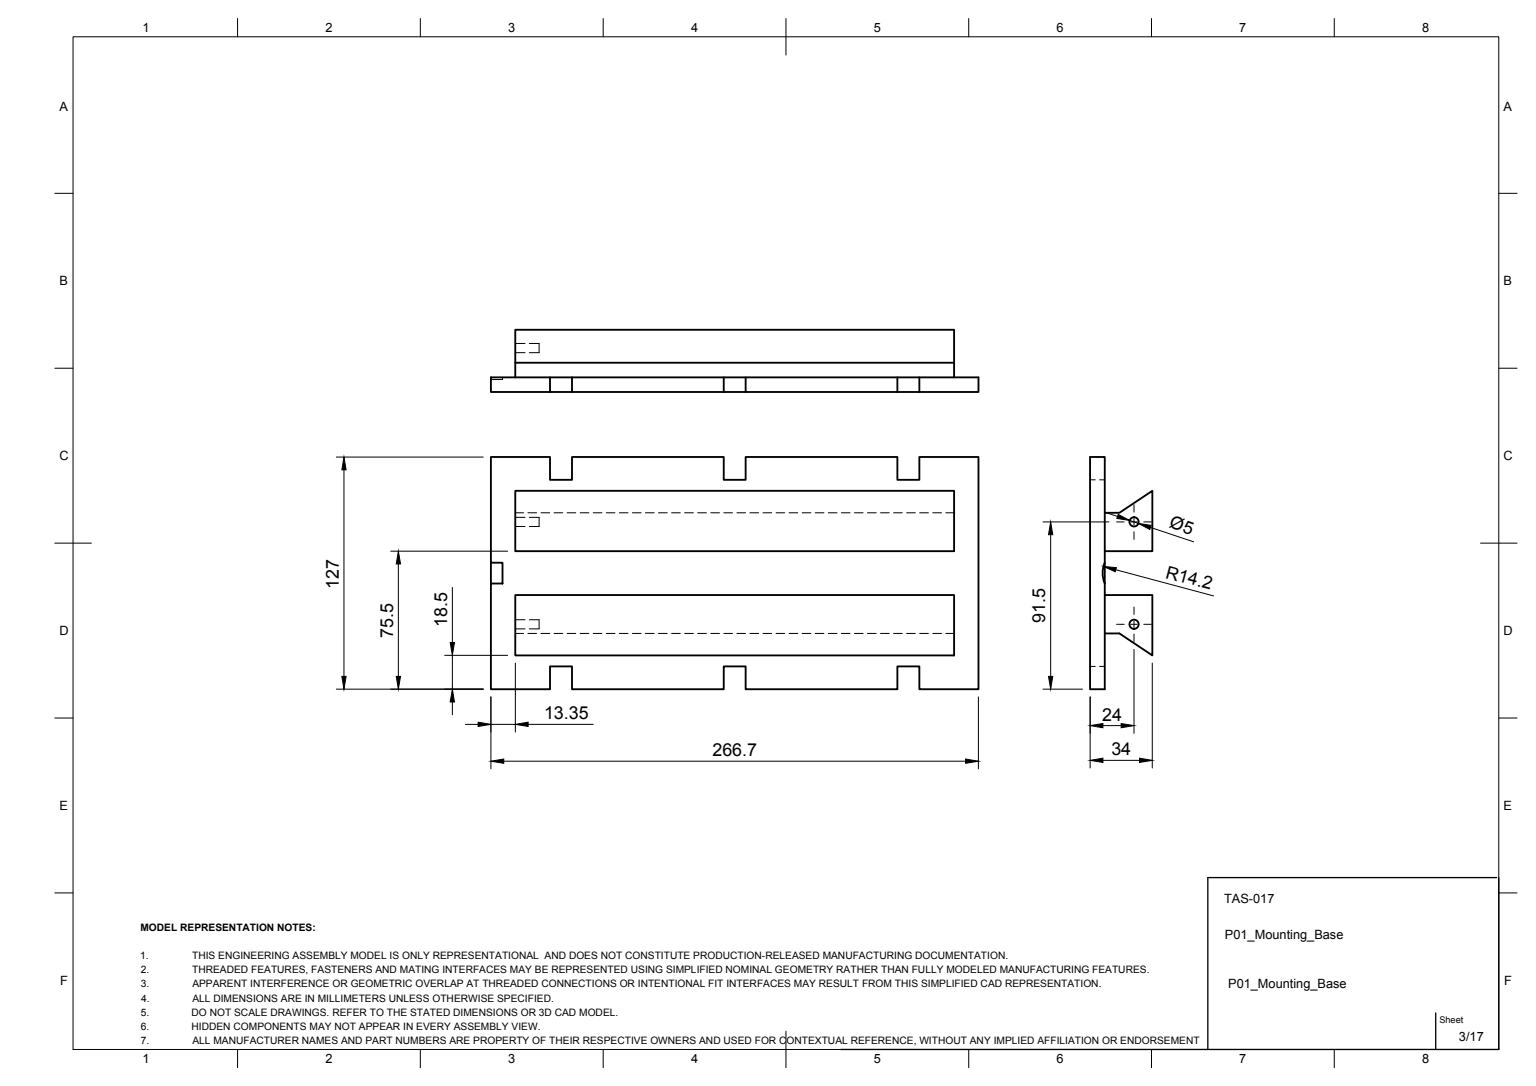
ISO-10303-21;
HEADER;
/* Generated by software containing ST-Developer
 * from STEP Tools, Inc. (www.steptools.com) 
 */

FILE_DESCRIPTION(
/* description */ ('STEP AP203'),
/* implementation_level */ '2;1');

FILE_NAME(
/* name */ 'P01_Mounting_Base.step',
/* time_stamp */ '2026-11-15T15:04:01-08:00',
/* author */ (''),
/* organization */ (''),
/* preprocessor_version */ 'ST-DEVELOPER v20.2',
/* originating_system */ 'Autodesk Translation Framework v15.17.0.0',
/* authorisation */ '');

FILE_SCHEMA (('AUTOMOTIVE_DESIGN { 1 0 10303 214 3 1 1 }'));
ENDSEC;

DATA;
#10=MECHANICAL_DESIGN_GEOMETRIC_PRESENTATION_REPRESENTATION('',(#276,#277,#278),#16598);
#204=SHAPE_REPRESENTATION_RELATIONSHIP('SRR','None',#16698,#228);
#228=ADVANCED_BREP_SHAPE_REPRESENTATION('',(#252),#16574);
#252=MANIFOLD_SOLID_BREP('Body1',#9787);
#276=STYLED_ITEM('',(#16828),#9252);
#277=STYLED_ITEM('',(#16828),#9258);
#278=STYLED_ITEM('',(#16827),#252);
#306=FACE_BOUND('',#1465,.T.);
#307=FACE_BOUND('',#1466,.T.);
#308=FACE_BOUND('',#1484,.T.);
#309=FACE_BOUND('',#1491,.T.);
#429=PLANE('',#10084);
#430=PLANE('',#10085);
#431=PLANE('',#10086);
#432=PLANE('',#10087);
#433=PLANE('',#10088);
#434=PLANE('',#10089);
#435=PLANE('',#10090);
#436=PLANE('',#10091);
#437=PLANE('',#10092);
#438=PLANE('',#10093);
#439=PLANE('',#10094);
#440=PLANE('',#10095);
#441=PLANE('',#10097);
#442=PLANE('',#10098);
#443=PLANE('',#10099);
#444=PLANE('',#10100);
#445=PLANE('',#10101);
#446=PLANE('',#10102);
#447=PLANE('',#10103);
#448=PLANE('',#10104);
#449=PLANE('',#10105);
#450=PLANE('',#10106);
#451=PLANE('',#10107);
#452=PLANE('',#10108);
#453=PLANE('',#10109);
#454=PLANE('',#10110);
#455=PLANE('',#10111);
#456=PLANE('',#10112);
#457=PLANE('',#10113);
#458=PLANE('',#10114);
#459=PLANE('',#10115);
#460=PLANE('',#10116);
#461=PLANE('',#10117);
#462=PLANE('',#10118);
#463=PLANE('',#10119);
#464=PLANE('',#10120);
#465=PLANE('',#10121);
#466=PLANE('',#10122);
#467=PLANE('',#10123);
#468=PLANE('',#10124);
#469=PLANE('',#10125);
#470=PLANE('',#10126);
#471=PLANE('',#10127);
#472=PLANE('',#10128);
#473=PLANE('',#10129);
#911=FACE_OUTER_BOUND('',#1462,.T.);
#912=FACE_OUTER_BOUND('',#1463,.T.);
#913=FACE_OUTER_BOUND('',#1464,.T.);
#914=FACE_OUTER_BOUND('',#1467,.T.);
#915=FACE_OUTER_BOUND('',#1468,.T.);
#916=FACE_OUTER_BOUND('',#1469,.T.);
#917=FACE_OUTER_BOUND('',#1470,.T.);
#918=FACE_OUTER_BOUND('',#1471,.T.);
#919=FACE_OUTER_BOUND('',#1472,.T.);
#920=FACE_OUTER_BOUND('',#1473,.T.);
#921=FACE_OUTER_BOUND('',#1474,.T.);
#922=FACE_OUTER_BOUND('',#1475,.T.);
#923=FACE_OUTER_BOUND('',#1476,.T.);
#924=FACE_OUTER_BOUND('',#1477,.T.);
#925=FACE_OUTER_BOUND('',#1478,.T.);
#926=FACE_OUTER_BOUND('',#1479,.T.);
#927=FACE_OUTER_BOUND('',#1480,.T.);
#928=FACE_OUTER_BOUND('',#1481,.T.);
#929=FACE_OUTER_BOUND('',#1482,.T.);
#930=FACE_OUTER_BOUND('',#1483,.T.);
#931=FACE_OUTER_BOUND('',#1485,.T.);
#932=FACE_OUTER_BOUND('',#1486,.T.);
#933=FACE_OUTER_BOUND('',#1487,.T.);
#934=FACE_OUTER_BOUND('',#1488,.T.);
#935=FACE_OUTER_BOUND('',#1489,.T.);
#936=FACE_OUTER_BOUND('',#1490,.T.);
#937=FACE_OUTER_BOUND('',#1492,.T.);
#938=FACE_OUTER_BOUND('',#1493,.T.);
#939=FACE_OUTER_BOUND('',#1494,.T.);
#940=FACE_OUTER_BOUND('',#1495,.T.);
#941=FACE_OUTER_BOUND('',#1496,.T.);
#942=FACE_OUTER_BOUND('',#1497,.T.);
#943=FACE_OUTER_BOUND('',#1498,.T.);
#944=FACE_OUTER_BOUND('',#1499,.T.);
#945=FACE_OUTER_BOUND('',#1500,.T.);
#946=FACE_OUTER_BOUND('',#1501,.T.);
#947=FACE_OUTER_BOUND('',#1502,.T.);
#948=FACE_OUTER_BOUND('',#1503,.T.);
#949=FACE_OUTER_BOUND('',#1504,.T.);
#950=FACE_OUTER_BOUND('',#1505,.T.);
#951=FACE_OUTER_BOUND('',#1506,.T.);
#952=FACE_OUTER_BOUND('',#1507,.T.);
#953=FACE_OUTER_BOUND('',#1508,.T.);
#954=FACE_OUTER_BOUND('',#1509,.T.);
#955=FACE_OUTER_BOUND('',#1510,.T.);
#956=FACE_OUTER_BOUND('',#1511,.T.);
#957=FACE_OUTER_BOUND('',#1512,.T.);
#958=FACE_OUTER_BOUND('',#1513,.T.);
#1462=EDGE_LOOP('',(#6597,#6598,#6599,#6600));
#1463=EDGE_LOOP('',(#6601,#6602,#6603,#6604));
#1464=EDGE_LOOP('',(#6605,#6606,#6607,#6608,#6609,#6610,#6611,#6612,#6613,
#6614,#6615,#6616,#6617,#6618,#6619,#6620,#6621,#6622,#6623,#6624,#6625,
#6626,#6627,#6628,#6629,#6630,#6631,#6632,#6633,#6634,#6635,#6636));
#1465=EDGE_LOOP('',(#6637,#6638,#6639,#6640));
#1466=EDGE_LOOP('',(#6641,#6642,#6643,#6644));
#1467=EDGE_LOOP('',(#6645,#6646,#6647,#6648));
#1468=EDGE_LOOP('',(#6649,#6650,#6651,#6652));
#1469=EDGE_LOOP('',(#6653,#6654,#6655,#6656));
#1470=EDGE_LOOP('',(#6657,#6658,#6659,#6660));
#1471=EDGE_LOOP('',(#6661,#6662,#6663,#6664));
#1472=EDGE_LOOP('',(#6665,#6666,#6667,#6668));
#1473=EDGE_LOOP('',(#6669,#6670,#6671,#6672));
#1474=EDGE_LOOP('',(#6673,#6674,#6675,#6676));
#1475=EDGE_LOOP('',(#6677,#6678,#6679,#6680,#6681,#6682,#6683,#6684,#6685,
#6686,#6687,#6688,#6689,#6690,#6691,#6692,#6693,#6694,#6695,#6696,#6697,
#6698,#6699,#6700,#6701,#6702,#6703,#6704));
#1476=EDGE_LOOP('',(#6705,#6706,#6707,#6708));
#1477=EDGE_LOOP('',(#6709,#6710,#6711,#6712,#6713,#6714));
#1478=EDGE_LOOP('',(#6715,#6716,#6717,#6718));
#1479=EDGE_LOOP('',(#6719,#6720,#6721,#6722));
#1480=EDGE_LOOP('',(#6723,#6724,#6725,#6726));
#1481=EDGE_LOOP('',(#6727,#6728,#6729,#6730));
#1482=EDGE_LOOP('',(#6731,#6732,#6733,#6734,#6735));
#1483=EDGE_LOOP('',(#6736,#6737,#6738,#6739,#6740));
#1484=EDGE_LOOP('',(#6741));
#1485=EDGE_LOOP('',(#6742,#6743,#6744,#6745));
#1486=EDGE_LOOP('',(#6746,#6747,#6748,#6749));
#1487=EDGE_LOOP('',(#6750,#6751,#6752,#6753));
#1488=EDGE_LOOP('',(#6754,#6755,#6756,#6757));
#1489=EDGE_LOOP('',(#6758,#6759,#6760,#6761,#6762));
#1490=EDGE_LOOP('',(#6763,#6764,#6765,#6766,#6767));
#1491=EDGE_LOOP('',(#6768));
#1492=EDGE_LOOP('',(#6769,#6770,#6771,#6772));
#1493=EDGE_LOOP('',(#6773,#6774,#6775,#6776));
#1494=EDGE_LOOP('',(#6777,#6778,#6779,#6780));
#1495=EDGE_LOOP('',(#6781,#6782,#6783,#6784));
#1496=EDGE_LOOP('',(#6785,#6786,#6787,#6788));
#1497=EDGE_LOOP('',(#6789,#6790,#6791,#6792));
#1498=EDGE_LOOP('',(#6793,#6794,#6795,#6796));
#1499=EDGE_LOOP('',(#6797,#6798,#6799,#6800));
#1500=EDGE_LOOP('',(#6801,#6802,#6803,#6804));
#1501=EDGE_LOOP('',(#6805,#6806,#6807,#6808));
#1502=EDGE_LOOP('',(#6809,#6810,#6811,#6812));
#1503=EDGE_LOOP('',(#6813,#6814,#6815,#6816));
#1504=EDGE_LOOP('',(#6817,#6818,#6819,#6820));
#1505=EDGE_LOOP('',(#6821,#6822,#6823,#6824));
#1506=EDGE_LOOP('',(#6825,#6826,#6827,#6828));
#1507=EDGE_LOOP('',(#6829,#6830,#6831,#6832));
#1508=EDGE_LOOP('',(#6833,#6834,#6835,#6836));
#1509=EDGE_LOOP('',(#6837,#6838,#6839,#6840));
#1510=EDGE_LOOP('',(#6841));
#1511=EDGE_LOOP('',(#6842));
#1512=EDGE_LOOP('',(#6843,#6844));
#1513=EDGE_LOOP('',(#6845,#6846,#6847,#6848));
#2136=LINE('',#13686,#3184);
#2137=LINE('',#13692,#3185);
#2138=LINE('',#13697,#3186);
#2139=LINE('',#13699,#3187);
#2140=LINE('',#13701,#3188);
#2141=LINE('',#13703,#3189);
#2142=LINE('',#13705,#3190);
#2143=LINE('',#13707,#3191);
#2144=LINE('',#13709,#3192);
#2145=LINE('',#13711,#3193);
#2146=LINE('',#13713,#3194);
#2147=LINE('',#13715,#3195);
#2148=LINE('',#13717,#3196);
#2149=LINE('',#13719,#3197);
#2150=LINE('',#13721,#3198);
#2151=LINE('',#13723,#3199);
#2152=LINE('',#13725,#3200);
#2153=LINE('',#13727,#3201);
#2154=LINE('',#13729,#3202);
#2155=LINE('',#13731,#3203);
#2156=LINE('',#13733,#3204);
#2157=LINE('',#13735,#3205);
#2158=LINE('',#13737,#3206);
#2159=LINE('',#13739,#3207);
#2160=LINE('',#13741,#3208);
#2161=LINE('',#13743,#3209);
#2162=LINE('',#13745,#3210);
#2163=LINE('',#13747,#3211);
#2164=LINE('',#13749,#3212);
#2165=LINE('',#13751,#3213);
#2166=LINE('',#13753,#3214);
#2167=LINE('',#13755,#3215);
#2168=LINE('',#13757,#3216);
#2169=LINE('',#13758,#3217);
#2170=LINE('',#13761,#3218);
#2171=LINE('',#13763,#3219);
#2172=LINE('',#13765,#3220);
#2173=LINE('',#13766,#3221);
#2174=LINE('',#13769,#3222);
#2175=LINE('',#13771,#3223);
#2176=LINE('',#13773,#3224);
#2177=LINE('',#13774,#3225);
#2178=LINE('',#13777,#3226);
#2179=LINE('',#13779,#3227);
#2180=LINE('',#13780,#3228);
#2181=LINE('',#13783,#3229);
#2182=LINE('',#13785,#3230);
#2183=LINE('',#13786,#3231);
#2184=LINE('',#13789,#3232);
#2185=LINE('',#13791,#3233);
#2186=LINE('',#13792,#3234);
#2187=LINE('',#13795,#3235);
#2188=LINE('',#13797,#3236);
#2189=LINE('',#13798,#3237);
#2190=LINE('',#13801,#3238);
#2191=LINE('',#13803,#3239);
#2192=LINE('',#13804,#3240);
#2193=LINE('',#13807,#3241);
#2194=LINE('',#13809,#3242);
#2195=LINE('',#13810,#3243);
#2196=LINE('',#13813,#3244);
#2197=LINE('',#13815,#3245);
#2198=LINE('',#13816,#3246);
#2199=LINE('',#13819,#3247);
#2200=LINE('',#13821,#3248);
#2201=LINE('',#13822,#3249);
#2202=LINE('',#13825,#3250);
#2203=LINE('',#13827,#3251);
#2204=LINE('',#13828,#3252);
#2205=LINE('',#13830,#3253);
#2206=LINE('',#13832,#3254);
#2207=LINE('',#13833,#3255);
#2208=LINE('',#13835,#3256);
#2209=LINE('',#13837,#3257);
#2210=LINE('',#13838,#3258);
#2211=LINE('',#13839,#3259);
#2212=LINE('',#13841,#3260);
#2213=LINE('',#13843,#3261);
#2214=LINE('',#13844,#3262);
#2215=LINE('',#13846,#3263);
#2216=LINE('',#13848,#3264);
#2217=LINE('',#13849,#3265);
#2218=LINE('',#13851,#3266);
#2219=LINE('',#13853,#3267);
#2220=LINE('',#13854,#3268);
#2221=LINE('',#13855,#3269);
#2222=LINE('',#13861,#3270);
#2223=LINE('',#13863,#3271);
#2224=LINE('',#13864,#3272);
#2225=LINE('',#13867,#3273);
#2226=LINE('',#13869,#3274);
#2227=LINE('',#13870,#3275);
#2228=LINE('',#13873,#3276);
#2229=LINE('',#13875,#3277);
#2230=LINE('',#13876,#3278);
#2231=LINE('',#13878,#3279);
#2232=LINE('',#13879,#3280);
#2233=LINE('',#13884,#3281);
#2234=LINE('',#13886,#3282);
#2235=LINE('',#13887,#3283);
#2236=LINE('',#13890,#3284);
#2237=LINE('',#13892,#3285);
#2238=LINE('',#13893,#3286);
#2239=LINE('',#13896,#3287);
#2240=LINE('',#13898,#3288);
#2241=LINE('',#13899,#3289);
#2242=LINE('',#13901,#3290);
#2243=LINE('',#13902,#3291);
#2244=LINE('',#13906,#3292);
#2245=LINE('',#13908,#3293);
#2246=LINE('',#13911,#3294);
#2247=LINE('',#13913,#3295);
#2248=LINE('',#13916,#3296);
#2249=LINE('',#13918,#3297);
#2250=LINE('',#13921,#3298);
#2251=LINE('',#13923,#3299);
#2252=LINE('',#13926,#3300);
#2253=LINE('',#13928,#3301);
#2254=LINE('',#13931,#3302);
#2255=LINE('',#13933,#3303);
#3184=VECTOR('',#10936,2.5);
#3185=VECTOR('',#10943,2.5);
#3186=VECTOR('',#10948,1000.);
#3187=VECTOR('',#10949,1000.);
#3188=VECTOR('',#10950,1000.);
#3189=VECTOR('',#10951,1000.);
#3190=VECTOR('',#10952,1000.);
#3191=VECTOR('',#10953,1000.);
#3192=VECTOR('',#10954,1000.);
#3193=VECTOR('',#10955,1000.);
#3194=VECTOR('',#10956,1000.);
#3195=VECTOR('',#10957,1000.);
#3196=VECTOR('',#10958,1000.);
#3197=VECTOR('',#10959,1000.);
#3198=VECTOR('',#10960,1000.);
#3199=VECTOR('',#10961,1000.);
#3200=VECTOR('',#10962,1000.);
#3201=VECTOR('',#10963,1000.);
#3202=VECTOR('',#10964,1000.);
#3203=VECTOR('',#10965,1000.);
#3204=VECTOR('',#10966,1000.);
#3205=VECTOR('',#10967,1000.);
#3206=VECTOR('',#10968,1000.);
#3207=VECTOR('',#10969,1000.);
#3208=VECTOR('',#10970,1000.);
#3209=VECTOR('',#10971,1000.);
#3210=VECTOR('',#10972,1000.);
#3211=VECTOR('',#10973,1000.);
#3212=VECTOR('',#10974,1000.);
#3213=VECTOR('',#10975,1000.);
#3214=VECTOR('',#10976,1000.);
#3215=VECTOR('',#10977,1000.);
#3216=VECTOR('',#10978,1000.);
#3217=VECTOR('',#10979,1000.);
#3218=VECTOR('',#10980,1000.);
#3219=VECTOR('',#10981,1000.);
#3220=VECTOR('',#10982,1000.);
#3221=VECTOR('',#10983,1000.);
#3222=VECTOR('',#10984,1000.);
#3223=VECTOR('',#10985,1000.);
#3224=VECTOR('',#10986,1000.);
#3225=VECTOR('',#10987,1000.);
#3226=VECTOR('',#10990,1000.);
#3227=VECTOR('',#10991,1000.);
#3228=VECTOR('',#10992,1000.);
#3229=VECTOR('',#10995,1000.);
#3230=VECTOR('',#10996,1000.);
#3231=VECTOR('',#10997,1000.);
#3232=VECTOR('',#11000,1000.);
#3233=VECTOR('',#11001,1000.);
#3234=VECTOR('',#11002,1000.);
#3235=VECTOR('',#11005,1000.);
#3236=VECTOR('',#11006,1000.);
#3237=VECTOR('',#11007,1000.);
#3238=VECTOR('',#11010,1000.);
#3239=VECTOR('',#11011,1000.);
#3240=VECTOR('',#11012,1000.);
#3241=VECTOR('',#11015,1000.);
#3242=VECTOR('',#11016,1000.);
#3243=VECTOR('',#11017,1000.);
#3244=VECTOR('',#11020,1000.);
#3245=VECTOR('',#11021,1000.);
#3246=VECTOR('',#11022,1000.);
#3247=VECTOR('',#11025,1000.);
#3248=VECTOR('',#11026,1000.);
#3249=VECTOR('',#11027,1000.);
#3250=VECTOR('',#11030,1000.);
#3251=VECTOR('',#11031,1000.);
#3252=VECTOR('',#11032,1000.);
#3253=VECTOR('',#11033,1000.);
#3254=VECTOR('',#11034,1000.);
#3255=VECTOR('',#11035,1000.);
#3256=VECTOR('',#11036,1000.);
#3257=VECTOR('',#11037,1000.);
#3258=VECTOR('',#11038,1000.);
#3259=VECTOR('',#11039,1000.);
#3260=VECTOR('',#11040,1000.);
#3261=VECTOR('',#11041,1000.);
#3262=VECTOR('',#11042,1000.);
#3263=VECTOR('',#11043,1000.);
#3264=VECTOR('',#11044,1000.);
#3265=VECTOR('',#11045,1000.);
#3266=VECTOR('',#11046,1000.);
#3267=VECTOR('',#11047,1000.);
#3268=VECTOR('',#11048,1000.);
#3269=VECTOR('',#11049,1000.);
#3270=VECTOR('',#11058,1000.);
#3271=VECTOR('',#11059,1000.);
#3272=VECTOR('',#11060,1000.);
#3273=VECTOR('',#11063,1000.);
#3274=VECTOR('',#11064,1000.);
#3275=VECTOR('',#11065,1000.);
#3276=VECTOR('',#11068,1000.);
#3277=VECTOR('',#11069,1000.);
#3278=VECTOR('',#11070,1000.);
#3279=VECTOR('',#11073,1000.);
#3280=VECTOR('',#11074,1000.);
#3281=VECTOR('',#11081,1000.);
#3282=VECTOR('',#11082,1000.);
#3283=VECTOR('',#11083,1000.);
#3284=VECTOR('',#11086,1000.);
#3285=VECTOR('',#11087,1000.);
#3286=VECTOR('',#11088,1000.);
#3287=VECTOR('',#11091,1000.);
#3288=VECTOR('',#11092,1000.);
#3289=VECTOR('',#11093,1000.);
#3290=VECTOR('',#11096,1000.);
#3291=VECTOR('',#11097,1000.);
#3292=VECTOR('',#11104,1000.);
#3293=VECTOR('',#11107,1000.);
#3294=VECTOR('',#11112,1000.);
#3295=VECTOR('',#11115,1000.);
#3296=VECTOR('',#11120,1000.);
#3297=VECTOR('',#11123,1000.);
#3298=VECTOR('',#11128,1000.);
#3299=VECTOR('',#11131,1000.);
#3300=VECTOR('',#11136,1000.);
#3301=VECTOR('',#11139,1000.);
#3302=VECTOR('',#11144,1000.);
#3303=VECTOR('',#11147,1000.);
#4232=CIRCLE('',#10079,2.5);
#4233=CIRCLE('',#10080,2.5);
#4234=CIRCLE('',#10082,2.5);
#4235=CIRCLE('',#10083,2.5);
#4236=CIRCLE('',#10096,14.2);
#4237=CIRCLE('',#10130,14.2);
#4455=VERTEX_POINT('',#13683);
#4456=VERTEX_POINT('',#13685);
#4457=VERTEX_POINT('',#13689);
#4458=VERTEX_POINT('',#13691);
#4459=VERTEX_POINT('',#13695);
#4460=VERTEX_POINT('',#13696);
#4461=VERTEX_POINT('',#13698);
#4462=VERTEX_POINT('',#13700);
#4463=VERTEX_POINT('',#13702);
#4464=VERTEX_POINT('',#13704);
#4465=VERTEX_POINT('',#13706);
#4466=VERTEX_POINT('',#13708);
#4467=VERTEX_POINT('',#13710);
#4468=VERTEX_POINT('',#13712);
#4469=VERTEX_POINT('',#13714);
#4470=VERTEX_POINT('',#13716);
#4471=VERTEX_POINT('',#13718);
#4472=VERTEX_POINT('',#13720);
#4473=VERTEX_POINT('',#13722);
#4474=VERTEX_POINT('',#13724);
#4475=VERTEX_POINT('',#13726);
#4476=VERTEX_POINT('',#13728);
#4477=VERTEX_POINT('',#13730);
#4478=VERTEX_POINT('',#13732);
#4479=VERTEX_POINT('',#13734);
#4480=VERTEX_POINT('',#13736);
#4481=VERTEX_POINT('',#13738);
#4482=VERTEX_POINT('',#13740);
#4483=VERTEX_POINT('',#13742);
#4484=VERTEX_POINT('',#13744);
#4485=VERTEX_POINT('',#13746);
#4486=VERTEX_POINT('',#13748);
#4487=VERTEX_POINT('',#13750);
#4488=VERTEX_POINT('',#13752);
#4489=VERTEX_POINT('',#13754);
#4490=VERTEX_POINT('',#13756);
#4491=VERTEX_POINT('',#13759);
#4492=VERTEX_POINT('',#13760);
#4493=VERTEX_POINT('',#13762);
#4494=VERTEX_POINT('',#13764);
#4495=VERTEX_POINT('',#13767);
#4496=VERTEX_POINT('',#13768);
#4497=VERTEX_POINT('',#13770);
#4498=VERTEX_POINT('',#13772);
#4499=VERTEX_POINT('',#13776);
#4500=VERTEX_POINT('',#13778);
#4501=VERTEX_POINT('',#13782);
#4502=VERTEX_POINT('',#13784);
#4503=VERTEX_POINT('',#13788);
#4504=VERTEX_POINT('',#13790);
#4505=VERTEX_POINT('',#13794);
#4506=VERTEX_POINT('',#13796);
#4507=VERTEX_POINT('',#13800);
#4508=VERTEX_POINT('',#13802);
#4509=VERTEX_POINT('',#13806);
#4510=VERTEX_POINT('',#13808);
#4511=VERTEX_POINT('',#13812);
#4512=VERTEX_POINT('',#13814);
#4513=VERTEX_POINT('',#13818);
#4514=VERTEX_POINT('',#13820);
#4515=VERTEX_POINT('',#13824);
#4516=VERTEX_POINT('',#13826);
#4517=VERTEX_POINT('',#13829);
#4518=VERTEX_POINT('',#13831);
#4519=VERTEX_POINT('',#13834);
#4520=VERTEX_POINT('',#13836);
#4521=VERTEX_POINT('',#13840);
#4522=VERTEX_POINT('',#13842);
#4523=VERTEX_POINT('',#13845);
#4524=VERTEX_POINT('',#13847);
#4525=VERTEX_POINT('',#13850);
#4526=VERTEX_POINT('',#13852);
#4527=VERTEX_POINT('',#13860);
#4528=VERTEX_POINT('',#13862);
#4529=VERTEX_POINT('',#13866);
#4530=VERTEX_POINT('',#13868);
#4531=VERTEX_POINT('',#13872);
#4532=VERTEX_POINT('',#13874);
#4533=VERTEX_POINT('',#13883);
#4534=VERTEX_POINT('',#13885);
#4535=VERTEX_POINT('',#13889);
#4536=VERTEX_POINT('',#13891);
#4537=VERTEX_POINT('',#13895);
#4538=VERTEX_POINT('',#13897);
#5311=EDGE_CURVE('',#4455,#4455,#4232,.T.);
#5312=EDGE_CURVE('',#4455,#4456,#2136,.T.);
#5313=EDGE_CURVE('',#4456,#4456,#4233,.T.);
#5314=EDGE_CURVE('',#4457,#4457,#4234,.T.);
#5315=EDGE_CURVE('',#4457,#4458,#2137,.T.);
#5316=EDGE_CURVE('',#4458,#4458,#4235,.T.);
#5317=EDGE_CURVE('',#4459,#4460,#2138,.T.);
#5318=EDGE_CURVE('',#4459,#4461,#2139,.T.);
#5319=EDGE_CURVE('',#4461,#4462,#2140,.T.);
#5320=EDGE_CURVE('',#4463,#4462,#2141,.T.);
#5321=EDGE_CURVE('',#4464,#4463,#2142,.T.);
#5322=EDGE_CURVE('',#4465,#4464,#2143,.T.);
#5323=EDGE_CURVE('',#4465,#4466,#2144,.T.);
#5324=EDGE_CURVE('',#4467,#4466,#2145,.T.);
#5325=EDGE_CURVE('',#4468,#4467,#2146,.T.);
#5326=EDGE_CURVE('',#4469,#4468,#2147,.T.);
#5327=EDGE_CURVE('',#4469,#4470,#2148,.T.);
#5328=EDGE_CURVE('',#4471,#4470,#2149,.T.);
#5329=EDGE_CURVE('',#4472,#4471,#2150,.T.);
#5330=EDGE_CURVE('',#4473,#4472,#2151,.T.);
#5331=EDGE_CURVE('',#4473,#4474,#2152,.T.);
#5332=EDGE_CURVE('',#4474,#4475,#2153,.T.);
#5333=EDGE_CURVE('',#4475,#4476,#2154,.T.);
#5334=EDGE_CURVE('',#4477,#4476,#2155,.T.);
#5335=EDGE_CURVE('',#4478,#4477,#2156,.T.);
#5336=EDGE_CURVE('',#4479,#4478,#2157,.T.);
#5337=EDGE_CURVE('',#4479,#4480,#2158,.T.);
#5338=EDGE_CURVE('',#4481,#4480,#2159,.T.);
#5339=EDGE_CURVE('',#4482,#4481,#2160,.T.);
#5340=EDGE_CURVE('',#4483,#4482,#2161,.T.);
#5341=EDGE_CURVE('',#4483,#4484,#2162,.T.);
#5342=EDGE_CURVE('',#4485,#4484,#2163,.T.);
#5343=EDGE_CURVE('',#4486,#4485,#2164,.T.);
#5344=EDGE_CURVE('',#4487,#4486,#2165,.T.);
#5345=EDGE_CURVE('',#4487,#4488,#2166,.T.);
#5346=EDGE_CURVE('',#4488,#4489,#2167,.T.);
#5347=EDGE_CURVE('',#4490,#4489,#2168,.T.);
#5348=EDGE_CURVE('',#4490,#4460,#2169,.T.);
#5349=EDGE_CURVE('',#4491,#4492,#2170,.T.);
#5350=EDGE_CURVE('',#4491,#4493,#2171,.T.);
#5351=EDGE_CURVE('',#4493,#4494,#2172,.T.);
#5352=EDGE_CURVE('',#4492,#4494,#2173,.T.);
#5353=EDGE_CURVE('',#4495,#4496,#2174,.T.);
#5354=EDGE_CURVE('',#4497,#4495,#2175,.T.);
#5355=EDGE_CURVE('',#4497,#4498,#2176,.T.);
#5356=EDGE_CURVE('',#4498,#4496,#2177,.T.);
#5357=EDGE_CURVE('',#4480,#4499,#2178,.T.);
#5358=EDGE_CURVE('',#4500,#4479,#2179,.T.);
#5359=EDGE_CURVE('',#4500,#4499,#2180,.T.);
#5360=EDGE_CURVE('',#4501,#4483,#2181,.T.);
#5361=EDGE_CURVE('',#4501,#4502,#2182,.T.);
#5362=EDGE_CURVE('',#4484,#4502,#2183,.T.);
#5363=EDGE_CURVE('',#4503,#4487,#2184,.T.);
#5364=EDGE_CURVE('',#4503,#4504,#2185,.T.);
#5365=EDGE_CURVE('',#4488,#4504,#2186,.T.);
#5366=EDGE_CURVE('',#4476,#4505,#2187,.T.);
#5367=EDGE_CURVE('',#4475,#4506,#2188,.T.);
#5368=EDGE_CURVE('',#4506,#4505,#2189,.T.);
#5369=EDGE_CURVE('',#4507,#4473,#2190,.T.);
#5370=EDGE_CURVE('',#4507,#4508,#2191,.T.);
#5371=EDGE_CURVE('',#4474,#4508,#2192,.T.);
#5372=EDGE_CURVE('',#4470,#4509,#2193,.T.);
#5373=EDGE_CURVE('',#4510,#4469,#2194,.T.);
#5374=EDGE_CURVE('',#4510,#4509,#2195,.T.);
#5375=EDGE_CURVE('',#4466,#4511,#2196,.T.);
#5376=EDGE_CURVE('',#4512,#4465,#2197,.T.);
#5377=EDGE_CURVE('',#4512,#4511,#2198,.T.);
#5378=EDGE_CURVE('',#4462,#4513,#2199,.T.);
#5379=EDGE_CURVE('',#4461,#4514,#2200,.T.);
#5380=EDGE_CURVE('',#4514,#4513,#2201,.T.);
#5381=EDGE_CURVE('',#4507,#4515,#2202,.T.);
#5382=EDGE_CURVE('',#4515,#4516,#2203,.T.);
#5383=EDGE_CURVE('',#4516,#4509,#2204,.T.);
#5384=EDGE_CURVE('',#4510,#4517,#2205,.T.);
#5385=EDGE_CURVE('',#4517,#4518,#2206,.T.);
#5386=EDGE_CURVE('',#4518,#4511,#2207,.T.);
#5387=EDGE_CURVE('',#4512,#4519,#2208,.T.);
#5388=EDGE_CURVE('',#4519,#4520,#2209,.T.);
#5389=EDGE_CURVE('',#4520,#4513,#2210,.T.);
#5390=EDGE_CURVE('',#4504,#4514,#2211,.T.);
#5391=EDGE_CURVE('',#4503,#4521,#2212,.T.);
#5392=EDGE_CURVE('',#4521,#4522,#2213,.T.);
#5393=EDGE_CURVE('',#4522,#4502,#2214,.T.);
#5394=EDGE_CURVE('',#4501,#4523,#2215,.T.);
#5395=EDGE_CURVE('',#4523,#4524,#2216,.T.);
#5396=EDGE_CURVE('',#4524,#4499,#2217,.T.);
#5397=EDGE_CURVE('',#4500,#4525,#2218,.T.);
#5398=EDGE_CURVE('',#4525,#4526,#2219,.T.);
#5399=EDGE_CURVE('',#4526,#4505,#2220,.T.);
#5400=EDGE_CURVE('',#4508,#4506,#2221,.T.);
#5401=EDGE_CURVE('',#4489,#4459,#4236,.T.);
#5402=EDGE_CURVE('',#4527,#4498,#2222,.T.);
#5403=EDGE_CURVE('',#4528,#4497,#2223,.T.);
#5404=EDGE_CURVE('',#4528,#4527,#2224,.T.);
#5405=EDGE_CURVE('',#4496,#4529,#2225,.T.);
#5406=EDGE_CURVE('',#4530,#4529,#2226,.T.);
#5407=EDGE_CURVE('',#4495,#4530,#2227,.T.);
#5408=EDGE_CURVE('',#4529,#4531,#2228,.T.);
#5409=EDGE_CURVE('',#4532,#4531,#2229,.T.);
#5410=EDGE_CURVE('',#4530,#4532,#2230,.T.);
#5411=EDGE_CURVE('',#4531,#4527,#2231,.T.);
#5412=EDGE_CURVE('',#4532,#4528,#2232,.T.);
#5413=EDGE_CURVE('',#4494,#4533,#2233,.T.);
#5414=EDGE_CURVE('',#4534,#4533,#2234,.T.);
#5415=EDGE_CURVE('',#4492,#4534,#2235,.T.);
#5416=EDGE_CURVE('',#4533,#4535,#2236,.T.);
#5417=EDGE_CURVE('',#4536,#4535,#2237,.T.);
#5418=EDGE_CURVE('',#4534,#4536,#2238,.T.);
#5419=EDGE_CURVE('',#4535,#4537,#2239,.T.);
#5420=EDGE_CURVE('',#4538,#4537,#2240,.T.);
#5421=EDGE_CURVE('',#4536,#4538,#2241,.T.);
#5422=EDGE_CURVE('',#4537,#4493,#2242,.T.);
#5423=EDGE_CURVE('',#4538,#4491,#2243,.T.);
#5424=EDGE_CURVE('',#4464,#4519,#2244,.T.);
#5425=EDGE_CURVE('',#4463,#4520,#2245,.T.);
#5426=EDGE_CURVE('',#4477,#4526,#2246,.T.);
#5427=EDGE_CURVE('',#4478,#4525,#2247,.T.);
#5428=EDGE_CURVE('',#4485,#4522,#2248,.T.);
#5429=EDGE_CURVE('',#4486,#4521,#2249,.T.);
#5430=EDGE_CURVE('',#4468,#4517,#2250,.T.);
#5431=EDGE_CURVE('',#4467,#4518,#2251,.T.);
#5432=EDGE_CURVE('',#4481,#4524,#2252,.T.);
#5433=EDGE_CURVE('',#4482,#4523,#2253,.T.);
#5434=EDGE_CURVE('',#4472,#4515,#2254,.T.);
#5435=EDGE_CURVE('',#4471,#4516,#2255,.T.);
#5436=EDGE_CURVE('',#4460,#4490,#4237,.T.);
#6597=ORIENTED_EDGE('',*,*,#5311,.T.);
#6598=ORIENTED_EDGE('',*,*,#5312,.T.);
#6599=ORIENTED_EDGE('',*,*,#5313,.T.);
#6600=ORIENTED_EDGE('',*,*,#5312,.F.);
#6601=ORIENTED_EDGE('',*,*,#5314,.T.);
#6602=ORIENTED_EDGE('',*,*,#5315,.T.);
#6603=ORIENTED_EDGE('',*,*,#5316,.F.);
#6604=ORIENTED_EDGE('',*,*,#5315,.F.);
#6605=ORIENTED_EDGE('',*,*,#5317,.F.);
#6606=ORIENTED_EDGE('',*,*,#5318,.T.);
#6607=ORIENTED_EDGE('',*,*,#5319,.T.);
#6608=ORIENTED_EDGE('',*,*,#5320,.F.);
#6609=ORIENTED_EDGE('',*,*,#5321,.F.);
#6610=ORIENTED_EDGE('',*,*,#5322,.F.);
#6611=ORIENTED_EDGE('',*,*,#5323,.T.);
#6612=ORIENTED_EDGE('',*,*,#5324,.F.);
#6613=ORIENTED_EDGE('',*,*,#5325,.F.);
#6614=ORIENTED_EDGE('',*,*,#5326,.F.);
#6615=ORIENTED_EDGE('',*,*,#5327,.T.);
#6616=ORIENTED_EDGE('',*,*,#5328,.F.);
#6617=ORIENTED_EDGE('',*,*,#5329,.F.);
#6618=ORIENTED_EDGE('',*,*,#5330,.F.);
#6619=ORIENTED_EDGE('',*,*,#5331,.T.);
#6620=ORIENTED_EDGE('',*,*,#5332,.T.);
#6621=ORIENTED_EDGE('',*,*,#5333,.T.);
#6622=ORIENTED_EDGE('',*,*,#5334,.F.);
#6623=ORIENTED_EDGE('',*,*,#5335,.F.);
#6624=ORIENTED_EDGE('',*,*,#5336,.F.);
#6625=ORIENTED_EDGE('',*,*,#5337,.T.);
#6626=ORIENTED_EDGE('',*,*,#5338,.F.);
#6627=ORIENTED_EDGE('',*,*,#5339,.F.);
#6628=ORIENTED_EDGE('',*,*,#5340,.F.);
#6629=ORIENTED_EDGE('',*,*,#5341,.T.);
#6630=ORIENTED_EDGE('',*,*,#5342,.F.);
#6631=ORIENTED_EDGE('',*,*,#5343,.F.);
#6632=ORIENTED_EDGE('',*,*,#5344,.F.);
#6633=ORIENTED_EDGE('',*,*,#5345,.T.);
#6634=ORIENTED_EDGE('',*,*,#5346,.T.);
#6635=ORIENTED_EDGE('',*,*,#5347,.F.);
#6636=ORIENTED_EDGE('',*,*,#5348,.T.);
#6637=ORIENTED_EDGE('',*,*,#5349,.F.);
#6638=ORIENTED_EDGE('',*,*,#5350,.T.);
#6639=ORIENTED_EDGE('',*,*,#5351,.T.);
#6640=ORIENTED_EDGE('',*,*,#5352,.F.);
#6641=ORIENTED_EDGE('',*,*,#5353,.F.);
#6642=ORIENTED_EDGE('',*,*,#5354,.F.);
#6643=ORIENTED_EDGE('',*,*,#5355,.T.);
#6644=ORIENTED_EDGE('',*,*,#5356,.T.);
#6645=ORIENTED_EDGE('',*,*,#5357,.F.);
#6646=ORIENTED_EDGE('',*,*,#5337,.F.);
#6647=ORIENTED_EDGE('',*,*,#5358,.F.);
#6648=ORIENTED_EDGE('',*,*,#5359,.T.);
#6649=ORIENTED_EDGE('',*,*,#5360,.F.);
#6650=ORIENTED_EDGE('',*,*,#5361,.T.);
#6651=ORIENTED_EDGE('',*,*,#5362,.F.);
#6652=ORIENTED_EDGE('',*,*,#5341,.F.);
#6653=ORIENTED_EDGE('',*,*,#5363,.F.);
#6654=ORIENTED_EDGE('',*,*,#5364,.T.);
#6655=ORIENTED_EDGE('',*,*,#5365,.F.);
#6656=ORIENTED_EDGE('',*,*,#5345,.F.);
#6657=ORIENTED_EDGE('',*,*,#5366,.F.);
#6658=ORIENTED_EDGE('',*,*,#5333,.F.);
#6659=ORIENTED_EDGE('',*,*,#5367,.T.);
#6660=ORIENTED_EDGE('',*,*,#5368,.T.);
#6661=ORIENTED_EDGE('',*,*,#5369,.F.);
#6662=ORIENTED_EDGE('',*,*,#5370,.T.);
#6663=ORIENTED_EDGE('',*,*,#5371,.F.);
#6664=ORIENTED_EDGE('',*,*,#5331,.F.);
#6665=ORIENTED_EDGE('',*,*,#5372,.F.);
#6666=ORIENTED_EDGE('',*,*,#5327,.F.);
#6667=ORIENTED_EDGE('',*,*,#5373,.F.);
#6668=ORIENTED_EDGE('',*,*,#5374,.T.);
#6669=ORIENTED_EDGE('',*,*,#5375,.F.);
#6670=ORIENTED_EDGE('',*,*,#5323,.F.);
#6671=ORIENTED_EDGE('',*,*,#5376,.F.);
#6672=ORIENTED_EDGE('',*,*,#5377,.T.);
#6673=ORIENTED_EDGE('',*,*,#5378,.F.);
#6674=ORIENTED_EDGE('',*,*,#5319,.F.);
#6675=ORIENTED_EDGE('',*,*,#5379,.T.);
#6676=ORIENTED_EDGE('',*,*,#5380,.T.);
#6677=ORIENTED_EDGE('',*,*,#5370,.F.);
#6678=ORIENTED_EDGE('',*,*,#5381,.T.);
#6679=ORIENTED_EDGE('',*,*,#5382,.T.);
#6680=ORIENTED_EDGE('',*,*,#5383,.T.);
#6681=ORIENTED_EDGE('',*,*,#5374,.F.);
#6682=ORIENTED_EDGE('',*,*,#5384,.T.);
#6683=ORIENTED_EDGE('',*,*,#5385,.T.);
#6684=ORIENTED_EDGE('',*,*,#5386,.T.);
#6685=ORIENTED_EDGE('',*,*,#5377,.F.);
#6686=ORIENTED_EDGE('',*,*,#5387,.T.);
#6687=ORIENTED_EDGE('',*,*,#5388,.T.);
#6688=ORIENTED_EDGE('',*,*,#5389,.T.);
#6689=ORIENTED_EDGE('',*,*,#5380,.F.);
#6690=ORIENTED_EDGE('',*,*,#5390,.F.);
#6691=ORIENTED_EDGE('',*,*,#5364,.F.);
#6692=ORIENTED_EDGE('',*,*,#5391,.T.);
#6693=ORIENTED_EDGE('',*,*,#5392,.T.);
#6694=ORIENTED_EDGE('',*,*,#5393,.T.);
#6695=ORIENTED_EDGE('',*,*,#5361,.F.);
#6696=ORIENTED_EDGE('',*,*,#5394,.T.);
#6697=ORIENTED_EDGE('',*,*,#5395,.T.);
#6698=ORIENTED_EDGE('',*,*,#5396,.T.);
#6699=ORIENTED_EDGE('',*,*,#5359,.F.);
#6700=ORIENTED_EDGE('',*,*,#5397,.T.);
#6701=ORIENTED_EDGE('',*,*,#5398,.T.);
#6702=ORIENTED_EDGE('',*,*,#5399,.T.);
#6703=ORIENTED_EDGE('',*,*,#5368,.F.);
#6704=ORIENTED_EDGE('',*,*,#5400,.F.);
#6705=ORIENTED_EDGE('',*,*,#5400,.T.);
#6706=ORIENTED_EDGE('',*,*,#5367,.F.);
#6707=ORIENTED_EDGE('',*,*,#5332,.F.);
#6708=ORIENTED_EDGE('',*,*,#5371,.T.);
#6709=ORIENTED_EDGE('',*,*,#5401,.F.);
#6710=ORIENTED_EDGE('',*,*,#5346,.F.);
#6711=ORIENTED_EDGE('',*,*,#5365,.T.);
#6712=ORIENTED_EDGE('',*,*,#5390,.T.);
#6713=ORIENTED_EDGE('',*,*,#5379,.F.);
#6714=ORIENTED_EDGE('',*,*,#5318,.F.);
#6715=ORIENTED_EDGE('',*,*,#5402,.T.);
#6716=ORIENTED_EDGE('',*,*,#5355,.F.);
#6717=ORIENTED_EDGE('',*,*,#5403,.F.);
#6718=ORIENTED_EDGE('',*,*,#5404,.T.);
#6719=ORIENTED_EDGE('',*,*,#5405,.T.);
#6720=ORIENTED_EDGE('',*,*,#5406,.F.);
#6721=ORIENTED_EDGE('',*,*,#5407,.F.);
#6722=ORIENTED_EDGE('',*,*,#5353,.T.);
#6723=ORIENTED_EDGE('',*,*,#5408,.T.);
#6724=ORIENTED_EDGE('',*,*,#5409,.F.);
#6725=ORIENTED_EDGE('',*,*,#5410,.F.);
#6726=ORIENTED_EDGE('',*,*,#5406,.T.);
#6727=ORIENTED_EDGE('',*,*,#5411,.T.);
#6728=ORIENTED_EDGE('',*,*,#5404,.F.);
#6729=ORIENTED_EDGE('',*,*,#5412,.F.);
#6730=ORIENTED_EDGE('',*,*,#5409,.T.);
#6731=ORIENTED_EDGE('',*,*,#5403,.T.);
#6732=ORIENTED_EDGE('',*,*,#5354,.T.);
#6733=ORIENTED_EDGE('',*,*,#5407,.T.);
#6734=ORIENTED_EDGE('',*,*,#5410,.T.);
#6735=ORIENTED_EDGE('',*,*,#5412,.T.);
#6736=ORIENTED_EDGE('',*,*,#5402,.F.);
#6737=ORIENTED_EDGE('',*,*,#5411,.F.);
#6738=ORIENTED_EDGE('',*,*,#5408,.F.);
#6739=ORIENTED_EDGE('',*,*,#5405,.F.);
#6740=ORIENTED_EDGE('',*,*,#5356,.F.);
#6741=ORIENTED_EDGE('',*,*,#5313,.F.);
#6742=ORIENTED_EDGE('',*,*,#5413,.T.);
#6743=ORIENTED_EDGE('',*,*,#5414,.F.);
#6744=ORIENTED_EDGE('',*,*,#5415,.F.);
#6745=ORIENTED_EDGE('',*,*,#5352,.T.);
#6746=ORIENTED_EDGE('',*,*,#5416,.T.);
#6747=ORIENTED_EDGE('',*,*,#5417,.F.);
#6748=ORIENTED_EDGE('',*,*,#5418,.F.);
#6749=ORIENTED_EDGE('',*,*,#5414,.T.);
#6750=ORIENTED_EDGE('',*,*,#5419,.T.);
#6751=ORIENTED_EDGE('',*,*,#5420,.F.);
#6752=ORIENTED_EDGE('',*,*,#5421,.F.);
#6753=ORIENTED_EDGE('',*,*,#5417,.T.);
#6754=ORIENTED_EDGE('',*,*,#5422,.T.);
#6755=ORIENTED_EDGE('',*,*,#5350,.F.);
#6756=ORIENTED_EDGE('',*,*,#5423,.F.);
#6757=ORIENTED_EDGE('',*,*,#5420,.T.);
#6758=ORIENTED_EDGE('',*,*,#5415,.T.);
#6759=ORIENTED_EDGE('',*,*,#5418,.T.);
#6760=ORIENTED_EDGE('',*,*,#5421,.T.);
#6761=ORIENTED_EDGE('',*,*,#5423,.T.);
#6762=ORIENTED_EDGE('',*,*,#5349,.T.);
#6763=ORIENTED_EDGE('',*,*,#5413,.F.);
#6764=ORIENTED_EDGE('',*,*,#5351,.F.);
#6765=ORIENTED_EDGE('',*,*,#5422,.F.);
#6766=ORIENTED_EDGE('',*,*,#5419,.F.);
#6767=ORIENTED_EDGE('',*,*,#5416,.F.);
#6768=ORIENTED_EDGE('',*,*,#5316,.T.);
#6769=ORIENTED_EDGE('',*,*,#5322,.T.);
#6770=ORIENTED_EDGE('',*,*,#5424,.T.);
#6771=ORIENTED_EDGE('',*,*,#5387,.F.);
#6772=ORIENTED_EDGE('',*,*,#5376,.T.);
#6773=ORIENTED_EDGE('',*,*,#5321,.T.);
#6774=ORIENTED_EDGE('',*,*,#5425,.T.);
#6775=ORIENTED_EDGE('',*,*,#5388,.F.);
#6776=ORIENTED_EDGE('',*,*,#5424,.F.);
#6777=ORIENTED_EDGE('',*,*,#5320,.T.);
#6778=ORIENTED_EDGE('',*,*,#5378,.T.);
#6779=ORIENTED_EDGE('',*,*,#5389,.F.);
#6780=ORIENTED_EDGE('',*,*,#5425,.F.);
#6781=ORIENTED_EDGE('',*,*,#5334,.T.);
#6782=ORIENTED_EDGE('',*,*,#5366,.T.);
#6783=ORIENTED_EDGE('',*,*,#5399,.F.);
#6784=ORIENTED_EDGE('',*,*,#5426,.F.);
#6785=ORIENTED_EDGE('',*,*,#5336,.T.);
#6786=ORIENTED_EDGE('',*,*,#5427,.T.);
#6787=ORIENTED_EDGE('',*,*,#5397,.F.);
#6788=ORIENTED_EDGE('',*,*,#5358,.T.);
#6789=ORIENTED_EDGE('',*,*,#5335,.T.);
#6790=ORIENTED_EDGE('',*,*,#5426,.T.);
#6791=ORIENTED_EDGE('',*,*,#5398,.F.);
#6792=ORIENTED_EDGE('',*,*,#5427,.F.);
#6793=ORIENTED_EDGE('',*,*,#5342,.T.);
#6794=ORIENTED_EDGE('',*,*,#5362,.T.);
#6795=ORIENTED_EDGE('',*,*,#5393,.F.);
#6796=ORIENTED_EDGE('',*,*,#5428,.F.);
#6797=ORIENTED_EDGE('',*,*,#5344,.T.);
#6798=ORIENTED_EDGE('',*,*,#5429,.T.);
#6799=ORIENTED_EDGE('',*,*,#5391,.F.);
#6800=ORIENTED_EDGE('',*,*,#5363,.T.);
#6801=ORIENTED_EDGE('',*,*,#5343,.T.);
#6802=ORIENTED_EDGE('',*,*,#5428,.T.);
#6803=ORIENTED_EDGE('',*,*,#5392,.F.);
#6804=ORIENTED_EDGE('',*,*,#5429,.F.);
#6805=ORIENTED_EDGE('',*,*,#5326,.T.);
#6806=ORIENTED_EDGE('',*,*,#5430,.T.);
#6807=ORIENTED_EDGE('',*,*,#5384,.F.);
#6808=ORIENTED_EDGE('',*,*,#5373,.T.);
#6809=ORIENTED_EDGE('',*,*,#5325,.T.);
#6810=ORIENTED_EDGE('',*,*,#5431,.T.);
#6811=ORIENTED_EDGE('',*,*,#5385,.F.);
#6812=ORIENTED_EDGE('',*,*,#5430,.F.);
#6813=ORIENTED_EDGE('',*,*,#5324,.T.);
#6814=ORIENTED_EDGE('',*,*,#5375,.T.);
#6815=ORIENTED_EDGE('',*,*,#5386,.F.);
#6816=ORIENTED_EDGE('',*,*,#5431,.F.);
#6817=ORIENTED_EDGE('',*,*,#5338,.T.);
#6818=ORIENTED_EDGE('',*,*,#5357,.T.);
#6819=ORIENTED_EDGE('',*,*,#5396,.F.);
#6820=ORIENTED_EDGE('',*,*,#5432,.F.);
#6821=ORIENTED_EDGE('',*,*,#5340,.T.);
#6822=ORIENTED_EDGE('',*,*,#5433,.T.);
#6823=ORIENTED_EDGE('',*,*,#5394,.F.);
#6824=ORIENTED_EDGE('',*,*,#5360,.T.);
#6825=ORIENTED_EDGE('',*,*,#5339,.T.);
#6826=ORIENTED_EDGE('',*,*,#5432,.T.);
#6827=ORIENTED_EDGE('',*,*,#5395,.F.);
#6828=ORIENTED_EDGE('',*,*,#5433,.F.);
#6829=ORIENTED_EDGE('',*,*,#5330,.T.);
#6830=ORIENTED_EDGE('',*,*,#5434,.T.);
#6831=ORIENTED_EDGE('',*,*,#5381,.F.);
#6832=ORIENTED_EDGE('',*,*,#5369,.T.);
#6833=ORIENTED_EDGE('',*,*,#5329,.T.);
#6834=ORIENTED_EDGE('',*,*,#5435,.T.);
#6835=ORIENTED_EDGE('',*,*,#5382,.F.);
#6836=ORIENTED_EDGE('',*,*,#5434,.F.);
#6837=ORIENTED_EDGE('',*,*,#5328,.T.);
#6838=ORIENTED_EDGE('',*,*,#5372,.T.);
#6839=ORIENTED_EDGE('',*,*,#5383,.F.);
#6840=ORIENTED_EDGE('',*,*,#5435,.F.);
#6841=ORIENTED_EDGE('',*,*,#5314,.F.);
#6842=ORIENTED_EDGE('',*,*,#5311,.F.);
#6843=ORIENTED_EDGE('',*,*,#5436,.F.);
#6844=ORIENTED_EDGE('',*,*,#5348,.F.);
#6845=ORIENTED_EDGE('',*,*,#5317,.T.);
#6846=ORIENTED_EDGE('',*,*,#5436,.T.);
#6847=ORIENTED_EDGE('',*,*,#5347,.T.);
#6848=ORIENTED_EDGE('',*,*,#5401,.T.);
#9169=CYLINDRICAL_SURFACE('',#10078,2.5);
#9170=CYLINDRICAL_SURFACE('',#10081,2.5);
#9171=CYLINDRICAL_SURFACE('',#10131,14.2);
#9236=ADVANCED_FACE('',(#911),#9169,.F.);
#9237=ADVANCED_FACE('',(#912),#9170,.F.);
#9238=ADVANCED_FACE('',(#913,#306,#307),#429,.F.);
#9239=ADVANCED_FACE('',(#914),#430,.F.);
#9240=ADVANCED_FACE('',(#915),#431,.F.);
#9241=ADVANCED_FACE('',(#916),#432,.F.);
#9242=ADVANCED_FACE('',(#917),#433,.F.);
#9243=ADVANCED_FACE('',(#918),#434,.F.);
#9244=ADVANCED_FACE('',(#919),#435,.F.);
#9245=ADVANCED_FACE('',(#920),#436,.F.);
#9246=ADVANCED_FACE('',(#921),#437,.F.);
#9247=ADVANCED_FACE('',(#922),#438,.T.);
#9248=ADVANCED_FACE('',(#923),#439,.F.);
#9249=ADVANCED_FACE('',(#924),#440,.F.);
#9250=ADVANCED_FACE('',(#925),#441,.F.);
#9251=ADVANCED_FACE('',(#926),#442,.F.);
#9252=ADVANCED_FACE('',(#927),#443,.F.);
#9253=ADVANCED_FACE('',(#928),#444,.F.);
#9254=ADVANCED_FACE('',(#929),#445,.T.);
#9255=ADVANCED_FACE('',(#930,#308),#446,.F.);
#9256=ADVANCED_FACE('',(#931),#447,.F.);
#9257=ADVANCED_FACE('',(#932),#448,.F.);
#9258=ADVANCED_FACE('',(#933),#449,.F.);
#9259=ADVANCED_FACE('',(#934),#450,.F.);
#9260=ADVANCED_FACE('',(#935),#451,.F.);
#9261=ADVANCED_FACE('',(#936,#309),#452,.T.);
#9262=ADVANCED_FACE('',(#937),#453,.T.);
#9263=ADVANCED_FACE('',(#938),#454,.T.);
#9264=ADVANCED_FACE('',(#939),#455,.T.);
#9265=ADVANCED_FACE('',(#940),#456,.T.);
#9266=ADVANCED_FACE('',(#941),#457,.T.);
#9267=ADVANCED_FACE('',(#942),#458,.T.);
#9268=ADVANCED_FACE('',(#943),#459,.T.);
#9269=ADVANCED_FACE('',(#944),#460,.T.);
#9270=ADVANCED_FACE('',(#945),#461,.T.);
#9271=ADVANCED_FACE('',(#946),#462,.T.);
#9272=ADVANCED_FACE('',(#947),#463,.T.);
#9273=ADVANCED_FACE('',(#948),#464,.T.);
#9274=ADVANCED_FACE('',(#949),#465,.T.);
#9275=ADVANCED_FACE('',(#950),#466,.T.);
#9276=ADVANCED_FACE('',(#951),#467,.T.);
#9277=ADVANCED_FACE('',(#952),#468,.T.);
#9278=ADVANCED_FACE('',(#953),#469,.T.);
#9279=ADVANCED_FACE('',(#954),#470,.T.);
#9280=ADVANCED_FACE('',(#955),#471,.F.);
#9281=ADVANCED_FACE('',(#956),#472,.F.);
#9282=ADVANCED_FACE('',(#957),#473,.F.);
#9283=ADVANCED_FACE('',(#958),#9171,.F.);
#9787=CLOSED_SHELL('',(#9236,#9237,#9238,#9239,#9240,#9241,#9242,#9243,
#9244,#9245,#9246,#9247,#9248,#9249,#9250,#9251,#9252,#9253,#9254,#9255,
#9256,#9257,#9258,#9259,#9260,#9261,#9262,#9263,#9264,#9265,#9266,#9267,
#9268,#9269,#9270,#9271,#9272,#9273,#9274,#9275,#9276,#9277,#9278,#9279,
#9280,#9281,#9282,#9283));
#10077=AXIS2_PLACEMENT_3D('',#13681,#10930,#10931);
#10078=AXIS2_PLACEMENT_3D('',#13682,#10932,#10933);
#10079=AXIS2_PLACEMENT_3D('',#13684,#10934,#10935);
#10080=AXIS2_PLACEMENT_3D('',#13687,#10937,#10938);
#10081=AXIS2_PLACEMENT_3D('',#13688,#10939,#10940);
#10082=AXIS2_PLACEMENT_3D('',#13690,#10941,#10942);
#10083=AXIS2_PLACEMENT_3D('',#13693,#10944,#10945);
#10084=AXIS2_PLACEMENT_3D('',#13694,#10946,#10947);
#10085=AXIS2_PLACEMENT_3D('',#13775,#10988,#10989);
#10086=AXIS2_PLACEMENT_3D('',#13781,#10993,#10994);
#10087=AXIS2_PLACEMENT_3D('',#13787,#10998,#10999);
#10088=AXIS2_PLACEMENT_3D('',#13793,#11003,#11004);
#10089=AXIS2_PLACEMENT_3D('',#13799,#11008,#11009);
#10090=AXIS2_PLACEMENT_3D('',#13805,#11013,#11014);
#10091=AXIS2_PLACEMENT_3D('',#13811,#11018,#11019);
#10092=AXIS2_PLACEMENT_3D('',#13817,#11023,#11024);
#10093=AXIS2_PLACEMENT_3D('',#13823,#11028,#11029);
#10094=AXIS2_PLACEMENT_3D('',#13856,#11050,#11051);
#10095=AXIS2_PLACEMENT_3D('',#13857,#11052,#11053);
#10096=AXIS2_PLACEMENT_3D('',#13858,#11054,#11055);
#10097=AXIS2_PLACEMENT_3D('',#13859,#11056,#11057);
#10098=AXIS2_PLACEMENT_3D('',#13865,#11061,#11062);
#10099=AXIS2_PLACEMENT_3D('',#13871,#11066,#11067);
#10100=AXIS2_PLACEMENT_3D('',#13877,#11071,#11072);
#10101=AXIS2_PLACEMENT_3D('',#13880,#11075,#11076);
#10102=AXIS2_PLACEMENT_3D('',#13881,#11077,#11078);
#10103=AXIS2_PLACEMENT_3D('',#13882,#11079,#11080);
#10104=AXIS2_PLACEMENT_3D('',#13888,#11084,#11085);
#10105=AXIS2_PLACEMENT_3D('',#13894,#11089,#11090);
#10106=AXIS2_PLACEMENT_3D('',#13900,#11094,#11095);
#10107=AXIS2_PLACEMENT_3D('',#13903,#11098,#11099);
#10108=AXIS2_PLACEMENT_3D('',#13904,#11100,#11101);
#10109=AXIS2_PLACEMENT_3D('',#13905,#11102,#11103);
#10110=AXIS2_PLACEMENT_3D('',#13907,#11105,#11106);
#10111=AXIS2_PLACEMENT_3D('',#13909,#11108,#11109);
#10112=AXIS2_PLACEMENT_3D('',#13910,#11110,#11111);
#10113=AXIS2_PLACEMENT_3D('',#13912,#11113,#11114);
#10114=AXIS2_PLACEMENT_3D('',#13914,#11116,#11117);
#10115=AXIS2_PLACEMENT_3D('',#13915,#11118,#11119);
#10116=AXIS2_PLACEMENT_3D('',#13917,#11121,#11122);
#10117=AXIS2_PLACEMENT_3D('',#13919,#11124,#11125);
#10118=AXIS2_PLACEMENT_3D('',#13920,#11126,#11127);
#10119=AXIS2_PLACEMENT_3D('',#13922,#11129,#11130);
#10120=AXIS2_PLACEMENT_3D('',#13924,#11132,#11133);
#10121=AXIS2_PLACEMENT_3D('',#13925,#11134,#11135);
#10122=AXIS2_PLACEMENT_3D('',#13927,#11137,#11138);
#10123=AXIS2_PLACEMENT_3D('',#13929,#11140,#11141);
#10124=AXIS2_PLACEMENT_3D('',#13930,#11142,#11143);
#10125=AXIS2_PLACEMENT_3D('',#13932,#11145,#11146);
#10126=AXIS2_PLACEMENT_3D('',#13934,#11148,#11149);
#10127=AXIS2_PLACEMENT_3D('',#13935,#11150,#11151);
#10128=AXIS2_PLACEMENT_3D('',#13936,#11152,#11153);
#10129=AXIS2_PLACEMENT_3D('',#13937,#11154,#11155);
#10130=AXIS2_PLACEMENT_3D('',#13938,#11156,#11157);
#10131=AXIS2_PLACEMENT_3D('',#13939,#11158,#11159);
#10930=DIRECTION('axis',(0.,0.,1.));
#10931=DIRECTION('refdir',(1.,0.,0.));
#10932=DIRECTION('center_axis',(-1.,0.,0.));
#10933=DIRECTION('ref_axis',(0.,0.,1.));
#10934=DIRECTION('center_axis',(1.,0.,0.));
#10935=DIRECTION('ref_axis',(0.,0.,-1.));
#10936=DIRECTION('',(-1.,0.,0.));
#10937=DIRECTION('center_axis',(-1.,0.,0.));
#10938=DIRECTION('ref_axis',(0.,0.,-1.));
#10939=DIRECTION('center_axis',(-1.,0.,0.));
#10940=DIRECTION('ref_axis',(0.,0.,1.));
#10941=DIRECTION('center_axis',(1.,0.,0.));
#10942=DIRECTION('ref_axis',(0.,0.,-1.));
#10943=DIRECTION('',(-1.,0.,0.));
#10944=DIRECTION('center_axis',(1.,0.,0.));
#10945=DIRECTION('ref_axis',(0.,0.,1.));
#10946=DIRECTION('center_axis',(0.,0.,-1.));
#10947=DIRECTION('ref_axis',(-1.,0.,0.));
#10948=DIRECTION('',(1.,0.,0.));
#10949=DIRECTION('',(0.,-1.,0.));
#10950=DIRECTION('',(1.,0.,0.));
#10951=DIRECTION('',(0.,-1.,0.));
#10952=DIRECTION('',(-1.,0.,0.));
#10953=DIRECTION('',(0.,1.,0.));
#10954=DIRECTION('',(1.,0.,0.));
#10955=DIRECTION('',(0.,-1.,0.));
#10956=DIRECTION('',(-1.,0.,0.));
#10957=DIRECTION('',(0.,1.,0.));
#10958=DIRECTION('',(1.,0.,0.));
#10959=DIRECTION('',(0.,-1.,0.));
#10960=DIRECTION('',(-1.,0.,0.));
#10961=DIRECTION('',(0.,1.,0.));
#10962=DIRECTION('',(1.,0.,0.));
#10963=DIRECTION('',(0.,1.,0.));
#10964=DIRECTION('',(-1.,0.,0.));
#10965=DIRECTION('',(0.,1.,0.));
#10966=DIRECTION('',(1.,0.,0.));
#10967=DIRECTION('',(0.,-1.,0.));
#10968=DIRECTION('',(-1.,0.,0.));
#10969=DIRECTION('',(0.,1.,0.));
#10970=DIRECTION('',(1.,0.,0.));
#10971=DIRECTION('',(0.,-1.,0.));
#10972=DIRECTION('',(-1.,0.,0.));
#10973=DIRECTION('',(0.,1.,0.));
#10974=DIRECTION('',(1.,0.,0.));
#10975=DIRECTION('',(0.,-1.,0.));
#10976=DIRECTION('',(-1.,0.,0.));
#10977=DIRECTION('',(0.,-1.,0.));
#10978=DIRECTION('',(-1.,0.,0.));
#10979=DIRECTION('',(0.,-1.,0.));
#10980=DIRECTION('',(0.,1.,0.));
#10981=DIRECTION('',(-1.,0.,0.));
#10982=DIRECTION('',(0.,1.,0.));
#10983=DIRECTION('',(-1.,0.,0.));
#10984=DIRECTION('',(-1.,0.,0.));
#10985=DIRECTION('',(0.,1.,0.));
#10986=DIRECTION('',(-1.,0.,0.));
#10987=DIRECTION('',(0.,1.,0.));
#10988=DIRECTION('center_axis',(0.,-1.,0.));
#10989=DIRECTION('ref_axis',(0.,0.,-1.));
#10990=DIRECTION('',(0.,0.,-1.));
#10991=DIRECTION('',(0.,0.,1.));
#10992=DIRECTION('',(-1.,0.,0.));
#10993=DIRECTION('center_axis',(0.,-1.,0.));
#10994=DIRECTION('ref_axis',(0.,0.,-1.));
#10995=DIRECTION('',(0.,0.,1.));
#10996=DIRECTION('',(-1.,0.,0.));
#10997=DIRECTION('',(0.,0.,-1.));
#10998=DIRECTION('center_axis',(0.,-1.,0.));
#10999=DIRECTION('ref_axis',(0.,0.,-1.));
#11000=DIRECTION('',(0.,0.,1.));
#11001=DIRECTION('',(-1.,0.,0.));
#11002=DIRECTION('',(0.,0.,-1.));
#11003=DIRECTION('center_axis',(0.,-1.,0.));
#11004=DIRECTION('ref_axis',(0.,0.,-1.));
#11005=DIRECTION('',(0.,0.,-1.));
#11006=DIRECTION('',(0.,0.,-1.));
#11007=DIRECTION('',(-1.,0.,0.));
#11008=DIRECTION('center_axis',(0.,1.,0.));
#11009=DIRECTION('ref_axis',(0.,0.,1.));
#11010=DIRECTION('',(0.,0.,1.));
#11011=DIRECTION('',(1.,0.,0.));
#11012=DIRECTION('',(0.,0.,-1.));
#11013=DIRECTION('center_axis',(0.,1.,0.));
#11014=DIRECTION('ref_axis',(0.,0.,1.));
#11015=DIRECTION('',(0.,0.,-1.));
#11016=DIRECTION('',(0.,0.,1.));
#11017=DIRECTION('',(1.,0.,0.));
#11018=DIRECTION('center_axis',(0.,1.,0.));
#11019=DIRECTION('ref_axis',(0.,0.,1.));
#11020=DIRECTION('',(0.,0.,-1.));
#11021=DIRECTION('',(0.,0.,1.));
#11022=DIRECTION('',(1.,0.,0.));
#11023=DIRECTION('center_axis',(0.,1.,0.));
#11024=DIRECTION('ref_axis',(0.,0.,1.));
#11025=DIRECTION('',(0.,0.,-1.));
#11026=DIRECTION('',(0.,0.,-1.));
#11027=DIRECTION('',(1.,0.,0.));
#11028=DIRECTION('center_axis',(0.,0.,-1.));
#11029=DIRECTION('ref_axis',(-1.,0.,0.));
#11030=DIRECTION('',(0.,1.,0.));
#11031=DIRECTION('',(-1.,0.,0.));
#11032=DIRECTION('',(0.,-1.,0.));
#11033=DIRECTION('',(0.,1.,0.));
#11034=DIRECTION('',(-1.,0.,0.));
#11035=DIRECTION('',(0.,-1.,0.));
#11036=DIRECTION('',(0.,1.,0.));
#11037=DIRECTION('',(-1.,0.,0.));
#11038=DIRECTION('',(0.,-1.,0.));
#11039=DIRECTION('',(0.,-1.,0.));
#11040=DIRECTION('',(0.,-1.,0.));
#11041=DIRECTION('',(1.,0.,0.));
#11042=DIRECTION('',(0.,1.,0.));
#11043=DIRECTION('',(0.,-1.,0.));
#11044=DIRECTION('',(1.,0.,0.));
#11045=DIRECTION('',(0.,1.,0.));
#11046=DIRECTION('',(0.,-1.,0.));
#11047=DIRECTION('',(1.,0.,0.));
#11048=DIRECTION('',(0.,1.,0.));
#11049=DIRECTION('',(0.,1.,0.));
#11050=DIRECTION('center_axis',(-1.,0.,0.));
#11051=DIRECTION('ref_axis',(0.,0.,1.));
#11052=DIRECTION('center_axis',(1.,0.,0.));
#11053=DIRECTION('ref_axis',(0.,0.,-1.));
#11054=DIRECTION('center_axis',(-1.,0.,0.));
#11055=DIRECTION('ref_axis',(0.,0.,-1.));
#11056=DIRECTION('center_axis',(0.,1.,0.));
#11057=DIRECTION('ref_axis',(0.,0.,1.));
#11058=DIRECTION('',(0.,0.,-1.));
#11059=DIRECTION('',(0.,0.,-1.));
#11060=DIRECTION('',(-1.,0.,0.));
#11061=DIRECTION('center_axis',(0.,-1.,0.));
#11062=DIRECTION('ref_axis',(0.,0.,-1.));
#11063=DIRECTION('',(0.,0.,1.));
#11064=DIRECTION('',(-1.,0.,0.));
#11065=DIRECTION('',(0.,0.,1.));
#11066=DIRECTION('center_axis',(0.,0.,-1.));
#11067=DIRECTION('ref_axis',(-1.,0.,0.));
#11068=DIRECTION('',(0.,-1.,0.));
#11069=DIRECTION('',(-1.,0.,0.));
#11070=DIRECTION('',(0.,-1.,0.));
#11071=DIRECTION('center_axis',(0.,0.832050294337844,0.554700196225229));
#11072=DIRECTION('ref_axis',(0.,-0.554700196225229,0.832050294337844));
#11073=DIRECTION('',(0.,0.554700196225229,-0.832050294337844));
#11074=DIRECTION('',(0.,0.554700196225229,-0.832050294337844));
#11075=DIRECTION('center_axis',(1.,0.,0.));
#11076=DIRECTION('ref_axis',(0.,0.,-1.));
#11077=DIRECTION('center_axis',(1.,0.,0.));
#11078=DIRECTION('ref_axis',(0.,0.,-1.));
#11079=DIRECTION('center_axis',(0.,-1.,0.));
#11080=DIRECTION('ref_axis',(0.,0.,-1.));
#11081=DIRECTION('',(0.,0.,1.));
#11082=DIRECTION('',(-1.,0.,0.));
#11083=DIRECTION('',(0.,0.,1.));
#11084=DIRECTION('center_axis',(0.,-0.832050294337844,0.554700196225229));
#11085=DIRECTION('ref_axis',(0.,-0.554700196225229,-0.832050294337844));
#11086=DIRECTION('',(0.,0.554700196225229,0.832050294337844));
#11087=DIRECTION('',(-1.,0.,0.));
#11088=DIRECTION('',(0.,0.554700196225229,0.832050294337844));
#11089=DIRECTION('center_axis',(0.,0.,-1.));
#11090=DIRECTION('ref_axis',(-1.,0.,0.));
#11091=DIRECTION('',(0.,-1.,0.));
#11092=DIRECTION('',(-1.,0.,0.));
#11093=DIRECTION('',(0.,-1.,0.));
#11094=DIRECTION('center_axis',(0.,1.,0.));
#11095=DIRECTION('ref_axis',(0.,0.,1.));
#11096=DIRECTION('',(0.,0.,-1.));
#11097=DIRECTION('',(0.,0.,-1.));
#11098=DIRECTION('center_axis',(-1.,0.,0.));
#11099=DIRECTION('ref_axis',(0.,0.,1.));
#11100=DIRECTION('center_axis',(-1.,0.,0.));
#11101=DIRECTION('ref_axis',(0.,0.,1.));
#11102=DIRECTION('center_axis',(-1.,0.,0.));
#11103=DIRECTION('ref_axis',(0.,0.,1.));
#11104=DIRECTION('',(0.,0.,-1.));
#11105=DIRECTION('center_axis',(0.,-1.,0.));
#11106=DIRECTION('ref_axis',(0.,0.,-1.));
#11107=DIRECTION('',(0.,0.,-1.));
#11108=DIRECTION('center_axis',(1.,0.,0.));
#11109=DIRECTION('ref_axis',(0.,0.,-1.));
#11110=DIRECTION('center_axis',(-1.,0.,0.));
#11111=DIRECTION('ref_axis',(0.,0.,1.));
#11112=DIRECTION('',(0.,0.,-1.));
#11113=DIRECTION('center_axis',(1.,0.,0.));
#11114=DIRECTION('ref_axis',(0.,0.,-1.));
#11115=DIRECTION('',(0.,0.,-1.));
#11116=DIRECTION('center_axis',(0.,1.,0.));
#11117=DIRECTION('ref_axis',(0.,0.,1.));
#11118=DIRECTION('center_axis',(-1.,0.,0.));
#11119=DIRECTION('ref_axis',(0.,0.,1.));
#11120=DIRECTION('',(0.,0.,-1.));
#11121=DIRECTION('center_axis',(1.,0.,0.));
#11122=DIRECTION('ref_axis',(0.,0.,-1.));
#11123=DIRECTION('',(0.,0.,-1.));
#11124=DIRECTION('center_axis',(0.,1.,0.));
#11125=DIRECTION('ref_axis',(0.,0.,1.));
#11126=DIRECTION('center_axis',(-1.,0.,0.));
#11127=DIRECTION('ref_axis',(0.,0.,1.));
#11128=DIRECTION('',(0.,0.,-1.));
#11129=DIRECTION('center_axis',(0.,-1.,0.));
#11130=DIRECTION('ref_axis',(0.,0.,-1.));
#11131=DIRECTION('',(0.,0.,-1.));
#11132=DIRECTION('center_axis',(1.,0.,0.));
#11133=DIRECTION('ref_axis',(0.,0.,-1.));
#11134=DIRECTION('center_axis',(-1.,0.,0.));
#11135=DIRECTION('ref_axis',(0.,0.,1.));
#11136=DIRECTION('',(0.,0.,-1.));
#11137=DIRECTION('center_axis',(1.,0.,0.));
#11138=DIRECTION('ref_axis',(0.,0.,-1.));
#11139=DIRECTION('',(0.,0.,-1.));
#11140=DIRECTION('center_axis',(0.,1.,0.));
#11141=DIRECTION('ref_axis',(0.,0.,1.));
#11142=DIRECTION('center_axis',(-1.,0.,0.));
#11143=DIRECTION('ref_axis',(0.,0.,1.));
#11144=DIRECTION('',(0.,0.,-1.));
#11145=DIRECTION('center_axis',(0.,-1.,0.));
#11146=DIRECTION('ref_axis',(0.,0.,-1.));
#11147=DIRECTION('',(0.,0.,-1.));
#11148=DIRECTION('center_axis',(1.,0.,0.));
#11149=DIRECTION('ref_axis',(0.,0.,-1.));
#11150=DIRECTION('center_axis',(1.,0.,0.));
#11151=DIRECTION('ref_axis',(0.,0.,-1.));
#11152=DIRECTION('center_axis',(1.,0.,0.));
#11153=DIRECTION('ref_axis',(0.,0.,-1.));
#11154=DIRECTION('center_axis',(1.,0.,0.));
#11155=DIRECTION('ref_axis',(0.,0.,-1.));
#11156=DIRECTION('center_axis',(1.,0.,0.));
#11157=DIRECTION('ref_axis',(0.,0.,-1.));
#11158=DIRECTION('center_axis',(-1.,0.,0.));
#11159=DIRECTION('ref_axis',(0.,-1.22464679914735E-16,-1.));
#13681=CARTESIAN_POINT('',(0.,0.,0.));
#13682=CARTESIAN_POINT('Origin',(-107.,-28.,24.));
#13683=CARTESIAN_POINT('',(-107.,-28.,21.5));
#13684=CARTESIAN_POINT('Origin',(-107.,-28.,24.));
#13685=CARTESIAN_POINT('',(-120.,-28.,21.5));
#13686=CARTESIAN_POINT('',(-107.,-28.,21.5));
#13687=CARTESIAN_POINT('Origin',(-120.,-28.,24.));
#13688=CARTESIAN_POINT('Origin',(-107.,28.,24.));
#13689=CARTESIAN_POINT('',(-107.,28.,21.5));
#13690=CARTESIAN_POINT('Origin',(-107.,28.,24.));
#13691=CARTESIAN_POINT('',(-120.,28.,21.5));
#13692=CARTESIAN_POINT('',(-107.,28.,21.5));
#13693=CARTESIAN_POINT('Origin',(-120.,28.,24.));
#13694=CARTESIAN_POINT('Origin',(0.,0.,8.));
#13695=CARTESIAN_POINT('',(-133.35,-5.71314274283428,8.));
#13696=CARTESIAN_POINT('',(-127.,-5.71314274283428,8.));
#13697=CARTESIAN_POINT('',(-127.,-5.71314274283428,8.));
#13698=CARTESIAN_POINT('',(-133.35,-63.5,8.));
#13699=CARTESIAN_POINT('',(-133.35,-63.5,8.));
#13700=CARTESIAN_POINT('',(-101.,-63.5,8.));
#13701=CARTESIAN_POINT('',(-133.35,-63.5,8.));
#13702=CARTESIAN_POINT('',(-101.,-51.,8.));
#13703=CARTESIAN_POINT('',(-101.,0.,8.));
#13704=CARTESIAN_POINT('',(-89.,-51.,8.));
#13705=CARTESIAN_POINT('',(0.,-51.,8.));
#13706=CARTESIAN_POINT('',(-89.,-63.5,8.));
#13707=CARTESIAN_POINT('',(-89.,0.,8.));
#13708=CARTESIAN_POINT('',(-6.00000000000001,-63.5,8.));
#13709=CARTESIAN_POINT('',(-133.35,-63.5,8.));
#13710=CARTESIAN_POINT('',(-6.,-51.,8.));
#13711=CARTESIAN_POINT('',(-6.,0.,8.));
#13712=CARTESIAN_POINT('',(6.,-51.,8.));
#13713=CARTESIAN_POINT('',(0.,-51.,8.));
#13714=CARTESIAN_POINT('',(6.00000000000001,-63.5,8.));
#13715=CARTESIAN_POINT('',(6.,0.,8.));
#13716=CARTESIAN_POINT('',(89.,-63.5,8.));
#13717=CARTESIAN_POINT('',(-133.35,-63.5,8.));
#13718=CARTESIAN_POINT('',(89.,-51.,8.));
#13719=CARTESIAN_POINT('',(89.,0.,8.));
#13720=CARTESIAN_POINT('',(101.,-51.,8.));
#13721=CARTESIAN_POINT('',(0.,-51.,8.));
#13722=CARTESIAN_POINT('',(101.,-63.5,8.));
#13723=CARTESIAN_POINT('',(101.,0.,8.));
#13724=CARTESIAN_POINT('',(133.35,-63.5,8.));
#13725=CARTESIAN_POINT('',(-133.35,-63.5,8.));
#13726=CARTESIAN_POINT('',(133.35,63.5,8.));
#13727=CARTESIAN_POINT('',(133.35,-63.5,8.));
#13728=CARTESIAN_POINT('',(101.,63.5,8.));
#13729=CARTESIAN_POINT('',(-133.35,63.5,8.));
#13730=CARTESIAN_POINT('',(101.,51.,8.));
#13731=CARTESIAN_POINT('',(101.,0.,8.));
#13732=CARTESIAN_POINT('',(89.,51.,8.));
#13733=CARTESIAN_POINT('',(0.,51.,8.));
#13734=CARTESIAN_POINT('',(89.,63.5,8.));
#13735=CARTESIAN_POINT('',(89.,0.,8.));
#13736=CARTESIAN_POINT('',(6.00000000000001,63.5,8.));
#13737=CARTESIAN_POINT('',(-133.35,63.5,8.));
#13738=CARTESIAN_POINT('',(6.,51.,8.));
#13739=CARTESIAN_POINT('',(6.,0.,8.));
#13740=CARTESIAN_POINT('',(-6.,51.,8.));
#13741=CARTESIAN_POINT('',(0.,51.,8.));
#13742=CARTESIAN_POINT('',(-6.00000000000001,63.5,8.));
#13743=CARTESIAN_POINT('',(-6.,0.,8.));
#13744=CARTESIAN_POINT('',(-89.,63.5,8.));
#13745=CARTESIAN_POINT('',(-133.35,63.5,8.));
#13746=CARTESIAN_POINT('',(-89.,51.,8.));
#13747=CARTESIAN_POINT('',(-89.,0.,8.));
#13748=CARTESIAN_POINT('',(-101.,51.,8.));
#13749=CARTESIAN_POINT('',(0.,51.,8.));
#13750=CARTESIAN_POINT('',(-101.,63.5,8.));
#13751=CARTESIAN_POINT('',(-101.,0.,8.));
#13752=CARTESIAN_POINT('',(-133.35,63.5,8.));
#13753=CARTESIAN_POINT('',(-133.35,63.5,8.));
#13754=CARTESIAN_POINT('',(-133.35,5.71314274283428,8.));
#13755=CARTESIAN_POINT('',(-133.35,-63.5,8.));
#13756=CARTESIAN_POINT('',(-127.,5.71314274283428,8.));
#13757=CARTESIAN_POINT('',(-127.,5.71314274283428,8.));
#13758=CARTESIAN_POINT('',(-127.,0.,8.));
#13759=CARTESIAN_POINT('',(120.,12.,8.));
#13760=CARTESIAN_POINT('',(120.,33.,8.));
#13761=CARTESIAN_POINT('',(120.,33.,8.));
#13762=CARTESIAN_POINT('',(-120.,12.,8.));
#13763=CARTESIAN_POINT('',(120.,12.,8.));
#13764=CARTESIAN_POINT('',(-120.,33.,8.));
#13765=CARTESIAN_POINT('',(-120.,33.,8.));
#13766=CARTESIAN_POINT('',(120.,33.,8.));
#13767=CARTESIAN_POINT('',(120.,-12.,8.));
#13768=CARTESIAN_POINT('',(-120.,-12.,8.));
#13769=CARTESIAN_POINT('',(120.,-12.,8.));
#13770=CARTESIAN_POINT('',(120.,-33.,8.));
#13771=CARTESIAN_POINT('',(120.,-33.,8.));
#13772=CARTESIAN_POINT('',(-120.,-33.,8.));
#13773=CARTESIAN_POINT('',(120.,-33.,8.));
#13774=CARTESIAN_POINT('',(-120.,-33.,8.));
#13775=CARTESIAN_POINT('Origin',(-133.35,63.5,8.));
#13776=CARTESIAN_POINT('',(6.,63.5,0.));
#13777=CARTESIAN_POINT('',(6.00000000000001,63.5,8.));
#13778=CARTESIAN_POINT('',(89.,63.5,0.));
#13779=CARTESIAN_POINT('',(89.,63.5,8.));
#13780=CARTESIAN_POINT('',(-133.35,63.5,0.));
#13781=CARTESIAN_POINT('Origin',(-133.35,63.5,8.));
#13782=CARTESIAN_POINT('',(-6.,63.5,0.));
#13783=CARTESIAN_POINT('',(-6.00000000000001,63.5,8.));
#13784=CARTESIAN_POINT('',(-89.,63.5,0.));
#13785=CARTESIAN_POINT('',(-133.35,63.5,0.));
#13786=CARTESIAN_POINT('',(-89.,63.5,8.));
#13787=CARTESIAN_POINT('Origin',(-133.35,63.5,8.));
#13788=CARTESIAN_POINT('',(-101.,63.5,0.));
#13789=CARTESIAN_POINT('',(-101.,63.5,8.));
#13790=CARTESIAN_POINT('',(-133.35,63.5,0.));
#13791=CARTESIAN_POINT('',(-133.35,63.5,0.));
#13792=CARTESIAN_POINT('',(-133.35,63.5,8.));
#13793=CARTESIAN_POINT('Origin',(-133.35,63.5,8.));
#13794=CARTESIAN_POINT('',(101.,63.5,0.));
#13795=CARTESIAN_POINT('',(101.,63.5,8.));
#13796=CARTESIAN_POINT('',(133.35,63.5,0.));
#13797=CARTESIAN_POINT('',(133.35,63.5,8.));
#13798=CARTESIAN_POINT('',(-133.35,63.5,0.));
#13799=CARTESIAN_POINT('Origin',(-133.35,-63.5,8.));
#13800=CARTESIAN_POINT('',(101.,-63.5,0.));
#13801=CARTESIAN_POINT('',(101.,-63.5,8.));
#13802=CARTESIAN_POINT('',(133.35,-63.5,0.));
#13803=CARTESIAN_POINT('',(-133.35,-63.5,0.));
#13804=CARTESIAN_POINT('',(133.35,-63.5,8.));
#13805=CARTESIAN_POINT('Origin',(-133.35,-63.5,8.));
#13806=CARTESIAN_POINT('',(89.,-63.5,0.));
#13807=CARTESIAN_POINT('',(89.,-63.5,8.));
#13808=CARTESIAN_POINT('',(6.,-63.5,0.));
#13809=CARTESIAN_POINT('',(6.00000000000001,-63.5,8.));
#13810=CARTESIAN_POINT('',(-133.35,-63.5,0.));
#13811=CARTESIAN_POINT('Origin',(-133.35,-63.5,8.));
#13812=CARTESIAN_POINT('',(-6.00000000000001,-63.5,0.));
#13813=CARTESIAN_POINT('',(-6.00000000000001,-63.5,8.));
#13814=CARTESIAN_POINT('',(-89.,-63.5,0.));
#13815=CARTESIAN_POINT('',(-89.,-63.5,8.));
#13816=CARTESIAN_POINT('',(-133.35,-63.5,0.));
#13817=CARTESIAN_POINT('Origin',(-133.35,-63.5,8.));
#13818=CARTESIAN_POINT('',(-101.,-63.5,0.));
#13819=CARTESIAN_POINT('',(-101.,-63.5,8.));
#13820=CARTESIAN_POINT('',(-133.35,-63.5,0.));
#13821=CARTESIAN_POINT('',(-133.35,-63.5,8.));
#13822=CARTESIAN_POINT('',(-133.35,-63.5,0.));
#13823=CARTESIAN_POINT('Origin',(0.,0.,0.));
#13824=CARTESIAN_POINT('',(101.,-51.,0.));
#13825=CARTESIAN_POINT('',(101.,0.,0.));
#13826=CARTESIAN_POINT('',(89.,-51.,0.));
#13827=CARTESIAN_POINT('',(0.,-51.,0.));
#13828=CARTESIAN_POINT('',(89.,0.,0.));
#13829=CARTESIAN_POINT('',(6.,-51.,0.));
#13830=CARTESIAN_POINT('',(6.,0.,0.));
#13831=CARTESIAN_POINT('',(-6.,-51.,0.));
#13832=CARTESIAN_POINT('',(0.,-51.,0.));
#13833=CARTESIAN_POINT('',(-6.,0.,0.));
#13834=CARTESIAN_POINT('',(-89.,-51.,0.));
#13835=CARTESIAN_POINT('',(-89.,0.,0.));
#13836=CARTESIAN_POINT('',(-101.,-51.,0.));
#13837=CARTESIAN_POINT('',(0.,-51.,0.));
#13838=CARTESIAN_POINT('',(-101.,0.,0.));
#13839=CARTESIAN_POINT('',(-133.35,-63.5,0.));
#13840=CARTESIAN_POINT('',(-101.,51.,0.));
#13841=CARTESIAN_POINT('',(-101.,0.,0.));
#13842=CARTESIAN_POINT('',(-89.,51.,0.));
#13843=CARTESIAN_POINT('',(0.,51.,0.));
#13844=CARTESIAN_POINT('',(-89.,0.,0.));
#13845=CARTESIAN_POINT('',(-6.,51.,0.));
#13846=CARTESIAN_POINT('',(-6.,0.,0.));
#13847=CARTESIAN_POINT('',(6.,51.,0.));
#13848=CARTESIAN_POINT('',(0.,51.,0.));
#13849=CARTESIAN_POINT('',(6.,0.,0.));
#13850=CARTESIAN_POINT('',(89.,51.,0.));
#13851=CARTESIAN_POINT('',(89.,0.,0.));
#13852=CARTESIAN_POINT('',(101.,51.,0.));
#13853=CARTESIAN_POINT('',(0.,51.,0.));
#13854=CARTESIAN_POINT('',(101.,0.,0.));
#13855=CARTESIAN_POINT('',(133.35,-63.5,0.));
#13856=CARTESIAN_POINT('Origin',(133.35,-63.5,8.));
#13857=CARTESIAN_POINT('Origin',(-133.35,-63.5,8.));
#13858=CARTESIAN_POINT('Origin',(-133.35,0.,21.));
#13859=CARTESIAN_POINT('Origin',(120.,-33.,16.));
#13860=CARTESIAN_POINT('',(-120.,-33.,16.));
#13861=CARTESIAN_POINT('',(-120.,-33.,16.));
#13862=CARTESIAN_POINT('',(120.,-33.,16.));
#13863=CARTESIAN_POINT('',(120.,-33.,16.));
#13864=CARTESIAN_POINT('',(120.,-33.,16.));
#13865=CARTESIAN_POINT('Origin',(120.,-12.,8.));
#13866=CARTESIAN_POINT('',(-120.,-12.,34.));
#13867=CARTESIAN_POINT('',(-120.,-12.,8.));
#13868=CARTESIAN_POINT('',(120.,-12.,34.));
#13869=CARTESIAN_POINT('',(120.,-12.,34.));
#13870=CARTESIAN_POINT('',(120.,-12.,8.));
#13871=CARTESIAN_POINT('Origin',(120.,-12.,34.));
#13872=CARTESIAN_POINT('',(-120.,-45.,34.));
#13873=CARTESIAN_POINT('',(-120.,-12.,34.));
#13874=CARTESIAN_POINT('',(120.,-45.,34.));
#13875=CARTESIAN_POINT('',(120.,-45.,34.));
#13876=CARTESIAN_POINT('',(120.,-12.,34.));
#13877=CARTESIAN_POINT('Origin',(120.,-45.,34.));
#13878=CARTESIAN_POINT('',(-120.,-45.,34.));
#13879=CARTESIAN_POINT('',(120.,-45.,34.));
#13880=CARTESIAN_POINT('Origin',(120.,0.,0.));
#13881=CARTESIAN_POINT('Origin',(-120.,0.,0.));
#13882=CARTESIAN_POINT('Origin',(120.,33.,16.));
#13883=CARTESIAN_POINT('',(-120.,33.,16.));
#13884=CARTESIAN_POINT('',(-120.,33.,16.));
#13885=CARTESIAN_POINT('',(120.,33.,16.));
#13886=CARTESIAN_POINT('',(120.,33.,16.));
#13887=CARTESIAN_POINT('',(120.,33.,16.));
#13888=CARTESIAN_POINT('Origin',(120.,45.,34.));
#13889=CARTESIAN_POINT('',(-120.,45.,34.));
#13890=CARTESIAN_POINT('',(-120.,45.,34.));
#13891=CARTESIAN_POINT('',(120.,45.,34.));
#13892=CARTESIAN_POINT('',(120.,45.,34.));
#13893=CARTESIAN_POINT('',(120.,45.,34.));
#13894=CARTESIAN_POINT('Origin',(120.,12.,34.));
#13895=CARTESIAN_POINT('',(-120.,12.,34.));
#13896=CARTESIAN_POINT('',(-120.,12.,34.));
#13897=CARTESIAN_POINT('',(120.,12.,34.));
#13898=CARTESIAN_POINT('',(120.,12.,34.));
#13899=CARTESIAN_POINT('',(120.,12.,34.));
#13900=CARTESIAN_POINT('Origin',(120.,12.,8.));
#13901=CARTESIAN_POINT('',(-120.,12.,8.));
#13902=CARTESIAN_POINT('',(120.,12.,8.));
#13903=CARTESIAN_POINT('Origin',(120.,0.,0.));
#13904=CARTESIAN_POINT('Origin',(-120.,0.,0.));
#13905=CARTESIAN_POINT('Origin',(-89.,-71.,9.));
#13906=CARTESIAN_POINT('',(-89.,-51.,9.));
#13907=CARTESIAN_POINT('Origin',(-101.,-51.,9.));
#13908=CARTESIAN_POINT('',(-101.,-51.,9.));
#13909=CARTESIAN_POINT('Origin',(-101.,-71.,9.));
#13910=CARTESIAN_POINT('Origin',(101.,51.,9.));
#13911=CARTESIAN_POINT('',(101.,51.,9.));
#13912=CARTESIAN_POINT('Origin',(89.,51.,9.));
#13913=CARTESIAN_POINT('',(89.,51.,9.));
#13914=CARTESIAN_POINT('Origin',(89.,51.,9.));
#13915=CARTESIAN_POINT('Origin',(-89.,51.,9.));
#13916=CARTESIAN_POINT('',(-89.,51.,9.));
#13917=CARTESIAN_POINT('Origin',(-101.,51.,9.));
#13918=CARTESIAN_POINT('',(-101.,51.,9.));
#13919=CARTESIAN_POINT('Origin',(-101.,51.,9.));
#13920=CARTESIAN_POINT('Origin',(6.,-71.,9.));
#13921=CARTESIAN_POINT('',(6.,-51.,9.));
#13922=CARTESIAN_POINT('Origin',(-6.,-51.,9.));
#13923=CARTESIAN_POINT('',(-6.,-51.,9.));
#13924=CARTESIAN_POINT('Origin',(-6.,-71.,9.));
#13925=CARTESIAN_POINT('Origin',(6.,51.,9.));
#13926=CARTESIAN_POINT('',(6.,51.,9.));
#13927=CARTESIAN_POINT('Origin',(-6.,51.,9.));
#13928=CARTESIAN_POINT('',(-6.,51.,9.));
#13929=CARTESIAN_POINT('Origin',(-6.,51.,9.));
#13930=CARTESIAN_POINT('Origin',(101.,-71.,9.));
#13931=CARTESIAN_POINT('',(101.,-51.,9.));
#13932=CARTESIAN_POINT('Origin',(89.,-51.,9.));
#13933=CARTESIAN_POINT('',(89.,-51.,9.));
#13934=CARTESIAN_POINT('Origin',(89.,-71.,9.));
#13935=CARTESIAN_POINT('Origin',(-107.,28.,24.));
#13936=CARTESIAN_POINT('Origin',(-107.,-28.,24.));
#13937=CARTESIAN_POINT('Origin',(-127.,0.,21.));
#13938=CARTESIAN_POINT('Origin',(-127.,0.,21.));
#13939=CARTESIAN_POINT('Origin',(-127.,0.,21.));
#16548=UNCERTAINTY_MEASURE_WITH_UNIT(LENGTH_MEASURE(0.01),#16599,
'DISTANCE_ACCURACY_VALUE',
'Maximum model space distance between geometric entities at asserted c
onnectivities');
#16572=UNCERTAINTY_MEASURE_WITH_UNIT(LENGTH_MEASURE(0.01),#16599,
'DISTANCE_ACCURACY_VALUE',
'Maximum model space distance between geometric entities at asserted c
onnectivities');
#16574=(
GEOMETRIC_REPRESENTATION_CONTEXT(3)
GLOBAL_UNCERTAINTY_ASSIGNED_CONTEXT((#16548))
GLOBAL_UNIT_ASSIGNED_CONTEXT((#16599,#16601,#16602))
REPRESENTATION_CONTEXT('','3D')
);
#16598=(
GEOMETRIC_REPRESENTATION_CONTEXT(3)
GLOBAL_UNCERTAINTY_ASSIGNED_CONTEXT((#16572))
GLOBAL_UNIT_ASSIGNED_CONTEXT((#16599,#16601,#16602))
REPRESENTATION_CONTEXT('','3D')
);
#16599=(
LENGTH_UNIT()
NAMED_UNIT(*)
SI_UNIT(.MILLI.,.METRE.)
);
#16601=(
NAMED_UNIT(*)
PLANE_ANGLE_UNIT()
SI_UNIT($,.RADIAN.)
);
#16602=(
NAMED_UNIT(*)
SI_UNIT($,.STERADIAN.)
SOLID_ANGLE_UNIT()
);
#16604=SHAPE_DEFINITION_REPRESENTATION(#16629,#16698);
#16629=PRODUCT_DEFINITION_SHAPE('',$,#16724);
#16698=SHAPE_REPRESENTATION('',(#10077),#16574);
#16722=PRODUCT_DEFINITION_CONTEXT('part definition',#16799,'design');
#16724=PRODUCT_DEFINITION('P01_Mounting_Base','P01_Mounting_Base',#16749,
#16722);
#16749=PRODUCT_DEFINITION_FORMATION('',$,#16802);
#16799=APPLICATION_CONTEXT(
'Core Data for Automotive Mechanical Design Process');
#16800=PRODUCT_CONTEXT('part definition',#16799,'mechanical');
#16802=PRODUCT('P01_Mounting_Base','P01_Mounting_Base',$,(#16800));
#16827=PRESENTATION_STYLE_ASSIGNMENT((#16836));
#16828=PRESENTATION_STYLE_ASSIGNMENT((#16837));
#16836=SURFACE_STYLE_USAGE(.BOTH.,#16845);
#16837=SURFACE_STYLE_USAGE(.BOTH.,#16846);
#16845=SURFACE_SIDE_STYLE('',(#16854));
#16846=SURFACE_SIDE_STYLE('',(#16855));
#16854=SURFACE_STYLE_FILL_AREA(#16863);
#16855=SURFACE_STYLE_FILL_AREA(#16864);
#16863=FILL_AREA_STYLE('Gray',(#16872));
#16864=FILL_AREA_STYLE('Opaque(147,158,163)',(#16873));
#16872=FILL_AREA_STYLE_COLOUR('Gray',#16881);
#16873=FILL_AREA_STYLE_COLOUR('Opaque(147,158,163)',#16882);
#16881=COLOUR_RGB('Gray',0.501960784313725,0.501960784313725,0.501960784313725);
#16882=COLOUR_RGB('Opaque(147,158,163)',0.576470588235294,0.619607843137255,
0.63921568627451);
ENDSEC;
END-ISO-10303-21;
